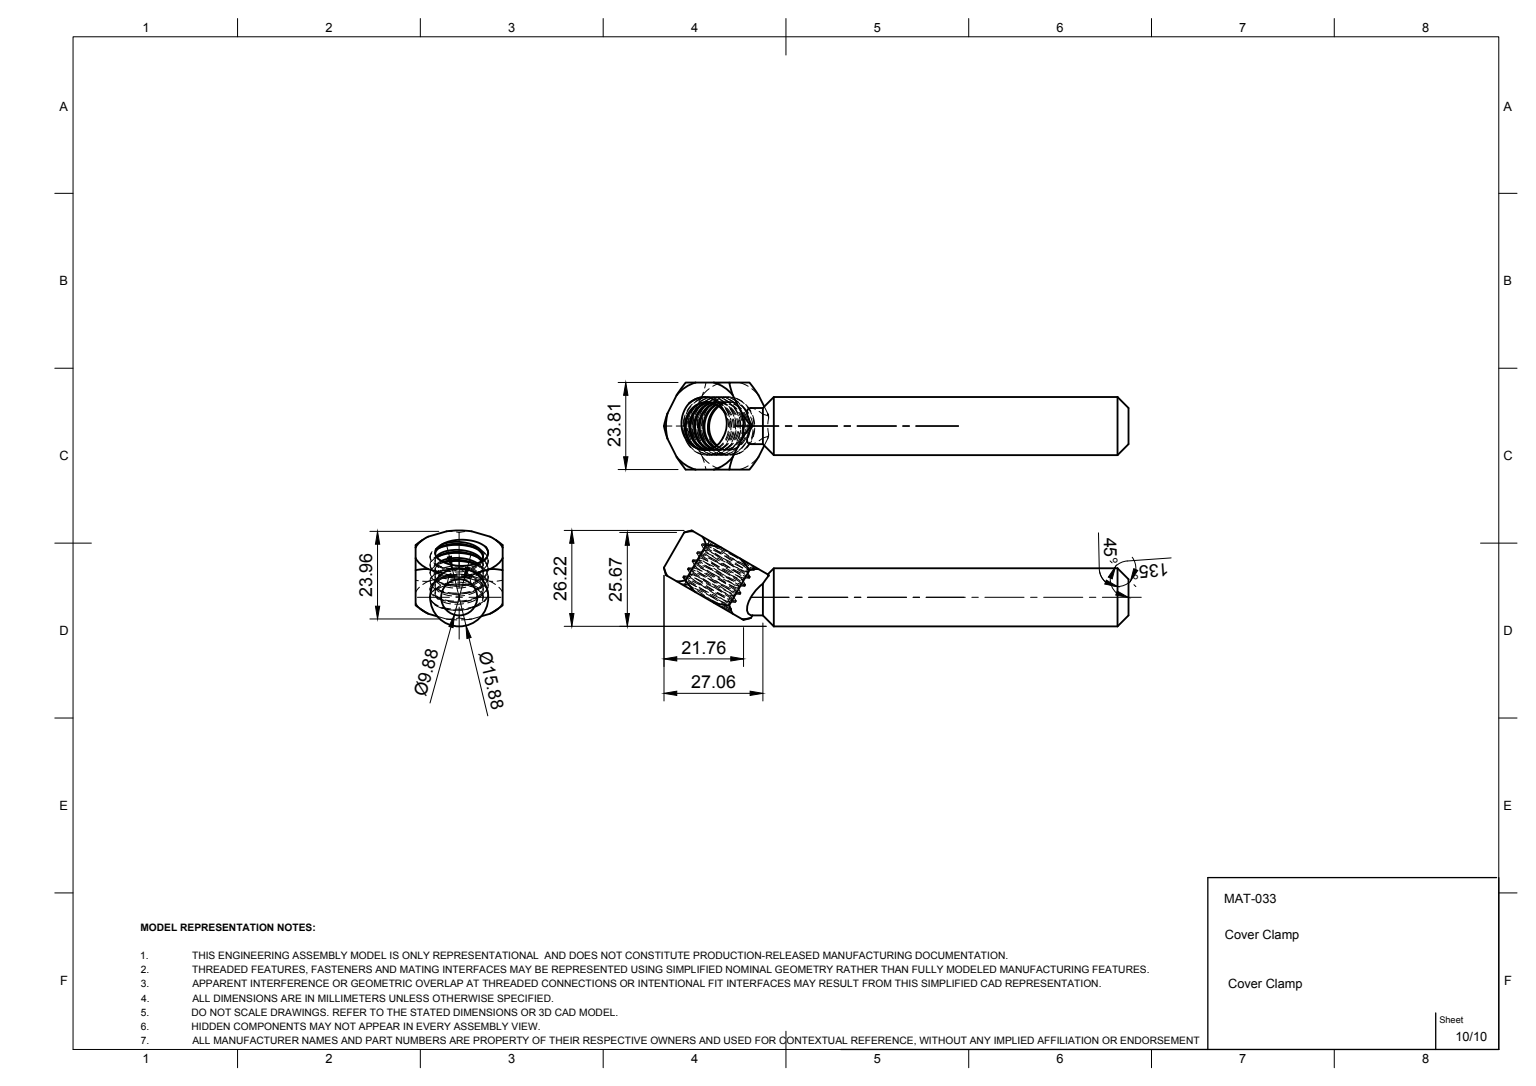
ISO-10303-21;
HEADER;
/* Generated by software containing ST-Developer
 * from STEP Tools, Inc. (www.steptools.com) 
 */

FILE_DESCRIPTION(
/* description */ ('STEP AP214'),
/* implementation_level */ '2;1');

FILE_NAME(
/* name */ 'Cover Clamp.step',
/* time_stamp */ '2026-11-14T07:13:32-08:00',
/* author */ (''),
/* organization */ (''),
/* preprocessor_version */ 'ST-DEVELOPER v20.2',
/* originating_system */ 'Autodesk Translation Framework v15.17.0.0',
/* authorisation */ '');

FILE_SCHEMA (('AUTOMOTIVE_DESIGN { 1 0 10303 214 3 1 1 }'));
ENDSEC;

DATA;
#10=MECHANICAL_DESIGN_GEOMETRIC_PRESENTATION_REPRESENTATION('',(#1323),#32903);
#315=(
BOUNDED_SURFACE()
B_SPLINE_SURFACE(1,2,((#30077,#30078,#30079,#30080,#30081,#30082,#30083,
#30084,#30085,#30086,#30087,#30088,#30089,#30090,#30091,#30092,#30093,#30094,
#30095,#30096,#30097,#30098,#30099,#30100,#30101,#30102,#30103,#30104,#30105,
#30106,#30107,#30108,#30109,#30110,#30111,#30112,#30113,#30114,#30115,#30116,
#30117,#30118,#30119,#30120,#30121,#30122,#30123,#30124,#30125,#30126,#30127,
#30128,#30129,#30130,#30131,#30132,#30133,#30134,#30135,#30136,#30137,#30138,
#30139,#30140,#30141,#30142,#30143,#30144,#30145,#30146,#30147,#30148,#30149,
#30150,#30151,#30152,#30153,#30154,#30155,#30156,#30157,#30158,#30159,#30160,
#30161,#30162,#30163,#30164,#30165,#30166,#30167,#30168,#30169,#30170,#30171,
#30172,#30173,#30174,#30175,#30176,#30177,#30178,#30179,#30180,#30181,#30182,
#30183,#30184,#30185,#30186,#30187,#30188,#30189,#30190,#30191,#30192,#30193,
#30194,#30195,#30196,#30197,#30198,#30199,#30200,#30201,#30202,#30203,#30204,
#30205,#30206,#30207,#30208,#30209,#30210,#30211,#30212,#30213),(#30214,
#30215,#30216,#30217,#30218,#30219,#30220,#30221,#30222,#30223,#30224,#30225,
#30226,#30227,#30228,#30229,#30230,#30231,#30232,#30233,#30234,#30235,#30236,
#30237,#30238,#30239,#30240,#30241,#30242,#30243,#30244,#30245,#30246,#30247,
#30248,#30249,#30250,#30251,#30252,#30253,#30254,#30255,#30256,#30257,#30258,
#30259,#30260,#30261,#30262,#30263,#30264,#30265,#30266,#30267,#30268,#30269,
#30270,#30271,#30272,#30273,#30274,#30275,#30276,#30277,#30278,#30279,#30280,
#30281,#30282,#30283,#30284,#30285,#30286,#30287,#30288,#30289,#30290,#30291,
#30292,#30293,#30294,#30295,#30296,#30297,#30298,#30299,#30300,#30301,#30302,
#30303,#30304,#30305,#30306,#30307,#30308,#30309,#30310,#30311,#30312,#30313,
#30314,#30315,#30316,#30317,#30318,#30319,#30320,#30321,#30322,#30323,#30324,
#30325,#30326,#30327,#30328,#30329,#30330,#30331,#30332,#30333,#30334,#30335,
#30336,#30337,#30338,#30339,#30340,#30341,#30342,#30343,#30344,#30345,#30346,
#30347,#30348,#30349,#30350)),.UNSPECIFIED.,.F.,.F.,.F.)
B_SPLINE_SURFACE_WITH_KNOTS((2,2),(3,2,2,2,2,2,2,2,2,2,2,2,2,2,2,2,2,2,
2,2,2,2,2,2,2,2,2,2,2,2,2,2,2,2,2,2,2,2,2,2,2,2,2,2,2,2,2,2,2,2,2,2,2,2,
2,2,2,2,2,2,2,2,2,2,2,2,2,2,3),(0.,1.),(0.,0.0142857142857143,0.0285714285714286,
0.0428571428571429,0.0571428571428571,0.0714285714285714,0.0857142857142857,
0.1,0.114285714285714,0.128571428571429,0.142857142857143,0.157142857142857,
0.171428571428571,0.185714285714286,0.2,0.214285714285714,0.228571428571429,
0.242857142857143,0.257142857142857,0.271428571428571,0.285714285714286,
0.3,0.314285714285714,0.328571428571429,0.342857142857143,0.357142857142857,
0.371428571428571,0.385714285714286,0.4,0.414285714285714,0.428571428571429,
0.442857142857143,0.457142857142857,0.471428571428571,0.485714285714286,
0.5,0.514285714285714,0.528571428571429,0.542857142857143,0.557142857142857,
0.571428571428571,0.585714285714286,0.6,0.614285714285714,0.628571428571429,
0.642857142857143,0.657142857142857,0.671428571428571,0.685714285714286,
0.7,0.714285714285714,0.728571428571429,0.742857142857143,0.757142857142857,
0.771428571428571,0.785714285714286,0.8,0.814285714285714,0.828571428571429,
0.842857142857143,0.857142857142857,0.871428571428571,0.885714285714286,
0.9,0.914285714285714,0.928571428571429,0.942857142857143,0.957142857142857,
0.961773175750461),.UNSPECIFIED.)
GEOMETRIC_REPRESENTATION_ITEM()
RATIONAL_B_SPLINE_SURFACE(((1.,0.951056516295154,1.,0.951056516295154,1.,
0.951056516295154,1.,0.951056516295154,1.,0.951056516295154,1.,0.951056516295154,
1.,0.951056516295154,1.,0.951056516295154,1.,0.951056516295154,1.,0.951056516295154,
1.,0.951056516295154,1.,0.951056516295154,1.,0.951056516295154,1.,0.951056516295154,
1.,0.951056516295154,1.,0.951056516295154,1.,0.951056516295154,1.,0.951056516295154,
1.,0.951056516295154,1.,0.951056516295154,1.,0.951056516295154,1.,0.951056516295154,
1.,0.951056516295154,1.,0.951056516295154,1.,0.951056516295154,1.,0.951056516295154,
1.,0.951056516295154,1.,0.951056516295154,1.,0.951056516295154,1.,0.951056516295154,
1.,0.951056516295154,1.,0.951056516295154,1.,0.951056516295154,1.,0.951056516295154,
1.,0.951056516295154,1.,0.951056516295154,1.,0.951056516295154,1.,0.951056516295154,
1.,0.951056516295154,1.,0.951056516295154,1.,0.951056516295154,1.,0.951056516295154,
1.,0.951056516295154,1.,0.951056516295154,1.,0.951056516295154,1.,0.951056516295154,
1.,0.951056516295154,1.,0.951056516295154,1.,0.951056516295154,1.,0.951056516295154,
1.,0.951056516295154,1.,0.951056516295154,1.,0.951056516295154,1.,0.951056516295154,
1.,0.951056516295154,1.,0.951056516295154,1.,0.951056516295154,1.,0.951056516295154,
1.,0.951056516295154,1.,0.951056516295154,1.,0.951056516295154,1.,0.951056516295154,
1.,0.951056516295154,1.,0.951056516295154,1.,0.951056516295154,1.,0.951056516295154,
1.,0.951056516295154,1.,0.984136325367634,0.978556192232199),(1.,0.951056516295154,
1.,0.951056516295154,1.,0.951056516295154,1.,0.951056516295154,1.,0.951056516295154,
1.,0.951056516295154,1.,0.951056516295154,1.,0.951056516295154,1.,0.951056516295154,
1.,0.951056516295154,1.,0.951056516295154,1.,0.951056516295154,1.,0.951056516295154,
1.,0.951056516295154,1.,0.951056516295154,1.,0.951056516295154,1.,0.951056516295154,
1.,0.951056516295154,1.,0.951056516295154,1.,0.951056516295154,1.,0.951056516295154,
1.,0.951056516295154,1.,0.951056516295154,1.,0.951056516295154,1.,0.951056516295154,
1.,0.951056516295154,1.,0.951056516295154,1.,0.951056516295154,1.,0.951056516295154,
1.,0.951056516295154,1.,0.951056516295154,1.,0.951056516295154,1.,0.951056516295154,
1.,0.951056516295154,1.,0.951056516295154,1.,0.951056516295154,1.,0.951056516295154,
1.,0.951056516295154,1.,0.951056516295154,1.,0.951056516295154,1.,0.951056516295154,
1.,0.951056516295154,1.,0.951056516295154,1.,0.951056516295154,1.,0.951056516295154,
1.,0.951056516295154,1.,0.951056516295154,1.,0.951056516295154,1.,0.951056516295154,
1.,0.951056516295154,1.,0.951056516295154,1.,0.951056516295154,1.,0.951056516295154,
1.,0.951056516295154,1.,0.951056516295154,1.,0.951056516295154,1.,0.951056516295154,
1.,0.951056516295154,1.,0.951056516295154,1.,0.951056516295154,1.,0.951056516295154,
1.,0.951056516295154,1.,0.951056516295154,1.,0.951056516295154,1.,0.951056516295154,
1.,0.951056516295154,1.,0.951056516295154,1.,0.984136325367634,0.978556192232199)))
REPRESENTATION_ITEM('')
SURFACE()
);
#316=(
BOUNDED_SURFACE()
B_SPLINE_SURFACE(1,2,((#30394,#30395,#30396,#30397,#30398,#30399,#30400,
#30401,#30402,#30403,#30404,#30405,#30406,#30407,#30408,#30409,#30410,#30411,
#30412,#30413,#30414,#30415,#30416,#30417,#30418,#30419,#30420,#30421,#30422,
#30423,#30424,#30425,#30426,#30427,#30428,#30429,#30430,#30431,#30432,#30433,
#30434,#30435,#30436,#30437,#30438,#30439,#30440,#30441,#30442,#30443,#30444,
#30445,#30446,#30447,#30448,#30449,#30450,#30451,#30452,#30453,#30454,#30455,
#30456,#30457,#30458,#30459,#30460,#30461,#30462,#30463,#30464,#30465,#30466,
#30467,#30468,#30469,#30470,#30471,#30472,#30473,#30474,#30475,#30476,#30477,
#30478,#30479,#30480,#30481,#30482,#30483,#30484,#30485,#30486,#30487,#30488,
#30489,#30490,#30491,#30492,#30493,#30494,#30495,#30496,#30497,#30498,#30499,
#30500,#30501,#30502,#30503,#30504,#30505,#30506,#30507,#30508,#30509,#30510,
#30511,#30512,#30513,#30514,#30515,#30516,#30517,#30518,#30519,#30520,#30521,
#30522,#30523,#30524,#30525,#30526,#30527,#30528,#30529,#30530),(#30531,
#30532,#30533,#30534,#30535,#30536,#30537,#30538,#30539,#30540,#30541,#30542,
#30543,#30544,#30545,#30546,#30547,#30548,#30549,#30550,#30551,#30552,#30553,
#30554,#30555,#30556,#30557,#30558,#30559,#30560,#30561,#30562,#30563,#30564,
#30565,#30566,#30567,#30568,#30569,#30570,#30571,#30572,#30573,#30574,#30575,
#30576,#30577,#30578,#30579,#30580,#30581,#30582,#30583,#30584,#30585,#30586,
#30587,#30588,#30589,#30590,#30591,#30592,#30593,#30594,#30595,#30596,#30597,
#30598,#30599,#30600,#30601,#30602,#30603,#30604,#30605,#30606,#30607,#30608,
#30609,#30610,#30611,#30612,#30613,#30614,#30615,#30616,#30617,#30618,#30619,
#30620,#30621,#30622,#30623,#30624,#30625,#30626,#30627,#30628,#30629,#30630,
#30631,#30632,#30633,#30634,#30635,#30636,#30637,#30638,#30639,#30640,#30641,
#30642,#30643,#30644,#30645,#30646,#30647,#30648,#30649,#30650,#30651,#30652,
#30653,#30654,#30655,#30656,#30657,#30658,#30659,#30660,#30661,#30662,#30663,
#30664,#30665,#30666,#30667)),.UNSPECIFIED.,.F.,.F.,.F.)
B_SPLINE_SURFACE_WITH_KNOTS((2,2),(3,2,2,2,2,2,2,2,2,2,2,2,2,2,2,2,2,2,
2,2,2,2,2,2,2,2,2,2,2,2,2,2,2,2,2,2,2,2,2,2,2,2,2,2,2,2,2,2,2,2,2,2,2,2,
2,2,2,2,2,2,2,2,2,2,2,2,2,2,3),(0.,1.),(0.,0.0142857142857143,0.0285714285714286,
0.0428571428571429,0.0571428571428571,0.0714285714285714,0.0857142857142857,
0.1,0.114285714285714,0.128571428571429,0.142857142857143,0.157142857142857,
0.171428571428571,0.185714285714286,0.2,0.214285714285714,0.228571428571429,
0.242857142857143,0.257142857142857,0.271428571428571,0.285714285714286,
0.3,0.314285714285714,0.328571428571429,0.342857142857143,0.357142857142857,
0.371428571428571,0.385714285714286,0.4,0.414285714285714,0.428571428571429,
0.442857142857143,0.457142857142857,0.471428571428571,0.485714285714286,
0.5,0.514285714285714,0.528571428571429,0.542857142857143,0.557142857142857,
0.571428571428571,0.585714285714286,0.6,0.614285714285714,0.628571428571429,
0.642857142857143,0.657142857142857,0.671428571428571,0.685714285714286,
0.7,0.714285714285714,0.728571428571429,0.742857142857143,0.757142857142857,
0.771428571428571,0.785714285714286,0.8,0.814285714285714,0.828571428571429,
0.842857142857143,0.857142857142857,0.871428571428571,0.885714285714286,
0.9,0.914285714285714,0.928571428571429,0.942857142857143,0.957142857142857,
0.961773131622773),.UNSPECIFIED.)
GEOMETRIC_REPRESENTATION_ITEM()
RATIONAL_B_SPLINE_SURFACE(((1.,0.951056516295154,1.,0.951056516295154,1.,
0.951056516295154,1.,0.951056516295154,1.,0.951056516295154,1.,0.951056516295154,
1.,0.951056516295154,1.,0.951056516295154,1.,0.951056516295154,1.,0.951056516295154,
1.,0.951056516295154,1.,0.951056516295154,1.,0.951056516295154,1.,0.951056516295154,
1.,0.951056516295154,1.,0.951056516295154,1.,0.951056516295154,1.,0.951056516295154,
1.,0.951056516295154,1.,0.951056516295154,1.,0.951056516295154,1.,0.951056516295154,
1.,0.951056516295154,1.,0.951056516295154,1.,0.951056516295154,1.,0.951056516295154,
1.,0.951056516295154,1.,0.951056516295154,1.,0.951056516295154,1.,0.951056516295154,
1.,0.951056516295154,1.,0.951056516295154,1.,0.951056516295154,1.,0.951056516295154,
1.,0.951056516295154,1.,0.951056516295154,1.,0.951056516295154,1.,0.951056516295154,
1.,0.951056516295154,1.,0.951056516295154,1.,0.951056516295154,1.,0.951056516295154,
1.,0.951056516295154,1.,0.951056516295154,1.,0.951056516295154,1.,0.951056516295154,
1.,0.951056516295154,1.,0.951056516295154,1.,0.951056516295154,1.,0.951056516295154,
1.,0.951056516295154,1.,0.951056516295154,1.,0.951056516295154,1.,0.951056516295154,
1.,0.951056516295154,1.,0.951056516295154,1.,0.951056516295154,1.,0.951056516295154,
1.,0.951056516295154,1.,0.951056516295154,1.,0.951056516295154,1.,0.951056516295154,
1.,0.951056516295154,1.,0.951056516295154,1.,0.951056516295154,1.,0.951056516295154,
1.,0.951056516295154,1.,0.98413647655103,0.978556298592283),(1.,0.951056516295154,
1.,0.951056516295154,1.,0.951056516295154,1.,0.951056516295154,1.,0.951056516295154,
1.,0.951056516295154,1.,0.951056516295154,1.,0.951056516295154,1.,0.951056516295154,
1.,0.951056516295154,1.,0.951056516295154,1.,0.951056516295154,1.,0.951056516295154,
1.,0.951056516295154,1.,0.951056516295154,1.,0.951056516295154,1.,0.951056516295154,
1.,0.951056516295154,1.,0.951056516295154,1.,0.951056516295154,1.,0.951056516295154,
1.,0.951056516295154,1.,0.951056516295154,1.,0.951056516295154,1.,0.951056516295154,
1.,0.951056516295154,1.,0.951056516295154,1.,0.951056516295154,1.,0.951056516295154,
1.,0.951056516295154,1.,0.951056516295154,1.,0.951056516295154,1.,0.951056516295154,
1.,0.951056516295154,1.,0.951056516295154,1.,0.951056516295154,1.,0.951056516295154,
1.,0.951056516295154,1.,0.951056516295154,1.,0.951056516295154,1.,0.951056516295154,
1.,0.951056516295154,1.,0.951056516295154,1.,0.951056516295154,1.,0.951056516295154,
1.,0.951056516295154,1.,0.951056516295154,1.,0.951056516295154,1.,0.951056516295154,
1.,0.951056516295154,1.,0.951056516295154,1.,0.951056516295154,1.,0.951056516295154,
1.,0.951056516295154,1.,0.951056516295154,1.,0.951056516295154,1.,0.951056516295154,
1.,0.951056516295154,1.,0.951056516295154,1.,0.951056516295154,1.,0.951056516295154,
1.,0.951056516295154,1.,0.951056516295154,1.,0.951056516295154,1.,0.951056516295154,
1.,0.951056516295154,1.,0.951056516295154,1.,0.98413647655103,0.978556298592283)))
REPRESENTATION_ITEM('')
SURFACE()
);
#388=B_SPLINE_CURVE_WITH_KNOTS('',3,(#29368,#29369,#29370,#29371,#29372,
#29373,#29374,#29375),.UNSPECIFIED.,.F.,.F.,(4,2,2,4),(9.99999998608377E-7,
0.266379961876312,0.531813270515335,0.536353198987997),.UNSPECIFIED.);
#389=B_SPLINE_CURVE_WITH_KNOTS('',3,(#29381,#29382,#29383,#29384,#29385,
#29386,#29387,#29388,#29389,#29390,#29391,#29392,#29393,#29394,#29395,#29396,
#29397,#29398,#29399,#29400,#29401,#29402,#29403,#29404,#29405,#29406,#29407,
#29408,#29409,#29410,#29411,#29412,#29413,#29414,#29415,#29416),
 .UNSPECIFIED.,.F.,.F.,(4,2,2,2,2,2,2,2,2,2,2,2,2,2,2,2,2,4),(22.8834714331197,
22.9155217152857,23.2228277353395,23.5358042737047,23.8457116148797,24.1541920344525,
24.4699609353675,24.7777751890622,25.0888369401879,25.401624583911,25.7090811724736,
26.0228085024749,26.332036183219,26.6411952597108,26.9577480048216,27.265398063477,
27.5359657548391,27.8035129251823),.UNSPECIFIED.);
#390=B_SPLINE_CURVE_WITH_KNOTS('',3,(#29418,#29419,#29420,#29421,#29422,
#29423,#29424,#29425,#29426,#29427,#29428,#29429,#29430,#29431,#29432,#29433,
#29434,#29435,#29436,#29437,#29438,#29439,#29440,#29441,#29442,#29443,#29444,
#29445,#29446,#29447,#29448,#29449,#29450,#29451,#29452,#29453),
 .UNSPECIFIED.,.F.,.F.,(4,2,2,2,2,2,2,2,2,2,2,2,2,2,2,2,2,4),(0.536353198987997,
0.844009151960195,1.15538573983787,1.46301980084842,1.7791232671795,2.0878690803984,
2.39732301411271,2.71061683058146,3.01790845407002,3.33114842108659,3.6418042399083,
3.94969512235302,4.26503959484436,4.57319165957025,4.88342264885394,5.19599272714235,
5.50322598252289,5.5439768298363),.UNSPECIFIED.);
#391=B_SPLINE_CURVE_WITH_KNOTS('',3,(#29458,#29459,#29460,#29461,#29462,
#29463,#29464,#29465,#29466,#29467,#29468,#29469,#29470,#29471,#29472,#29473,
#29474,#29475,#29476,#29477,#29478,#29479,#29480,#29481,#29482,#29483,#29484,
#29485,#29486,#29487,#29488,#29489,#29490,#29491,#29492,#29493),
 .UNSPECIFIED.,.F.,.F.,(4,2,2,2,2,2,2,2,2,2,2,2,2,2,2,2,2,4),(17.8745023500825,
17.9426329487553,18.2502173426604,18.5619029033133,18.8737351023357,19.1814304857963,
19.4958276241938,19.8045434042373,20.1142954786953,20.4295794098716,20.7369298255106,
21.0492181265779,21.360004308523,21.6679912272627,21.983034000075,22.2912070574588,
22.601577623486,22.8834714331197),.UNSPECIFIED.);
#392=B_SPLINE_CURVE_WITH_KNOTS('',3,(#29494,#29495,#29496,#29497,#29498,
#29499,#29500,#29501,#29502,#29503,#29504,#29505,#29506,#29507,#29508,#29509,
#29510,#29511,#29512,#29513,#29514,#29515,#29516,#29517,#29518,#29519,#29520,
#29521,#29522,#29523,#29524,#29525,#29526,#29527,#29528,#29529),
 .UNSPECIFIED.,.F.,.F.,(4,2,2,2,2,2,2,2,2,2,2,2,2,2,2,2,2,4),(5.5439768298363,
5.8177146782931,6.12771125014353,6.43605042222614,6.75070419648573,7.05845758227753,
7.36965133741442,7.68157100910749,7.98894019875319,8.30483846765822,8.61425879594142,
8.92321980318127,9.23727438509702,9.54483326301095,9.85713746478567,10.1685030197442,
10.4761899795599,10.5523964499815),.UNSPECIFIED.);
#393=B_SPLINE_CURVE_WITH_KNOTS('',3,(#29534,#29535,#29536,#29537,#29538,
#29539,#29540,#29541,#29542,#29543,#29544,#29545,#29546,#29547,#29548,#29549,
#29550,#29551,#29552,#29553,#29554,#29555,#29556,#29557,#29558,#29559,#29560,
#29561,#29562,#29563,#29564,#29565,#29566,#29567,#29568,#29569),
 .UNSPECIFIED.,.F.,.F.,(4,2,2,2,2,2,2,2,2,2,2,2,2,2,2,2,2,4),(12.8667522473679,
12.9699770959428,13.2778173876454,13.5932720524022,13.9015013605794,14.2087341790668,
14.5215936127585,14.8314800687057,15.1398530720226,15.4555019865385,15.7632628653506,
16.0742081083735,16.3869911773338,16.694362346664,17.0079690989337,17.3171627992321,
17.6262033882063,17.8745023500825),.UNSPECIFIED.);
#394=B_SPLINE_CURVE_WITH_KNOTS('',3,(#29570,#29571,#29572,#29573,#29574,
#29575,#29576,#29577,#29578,#29579,#29580,#29581,#29582,#29583,#29584,#29585,
#29586,#29587,#29588,#29589,#29590,#29591,#29592,#29593,#29594,#29595,#29596,
#29597,#29598,#29599,#29600,#29601,#29602,#29603,#29604,#29605),
 .UNSPECIFIED.,.F.,.F.,(4,2,2,2,2,2,2,2,2,2,2,2,2,2,2,2,2,4),(10.5523964499815,
10.7922801625917,11.1010192151014,11.4105628806873,11.7238453805044,12.0311675378644,
12.344531578361,12.655179957593,12.9631375944165,13.2784727772684,13.5866311789278,
13.8969661452367,14.2099076813701,14.5197896220926,14.8282363019679,15.1439697099529,
15.4517555491791,15.5606140240025),.UNSPECIFIED.);
#395=B_SPLINE_CURVE_WITH_KNOTS('',3,(#29610,#29611,#29612,#29613,#29614,
#29615,#29616,#29617,#29618,#29619,#29620,#29621,#29622,#29623,#29624,#29625,
#29626,#29627,#29628,#29629,#29630,#29631,#29632,#29633,#29634,#29635,#29636,
#29637,#29638,#29639,#29640,#29641,#29642,#29643,#29644,#29645),
 .UNSPECIFIED.,.F.,.F.,(4,2,2,2,2,2,2,2,2,2,2,2,2,2,2,2,2,4),(7.85839646972881,
7.99675908034552,8.30409236965206,8.61967918417833,8.92922883729377,9.23804955367523,
9.55223789637168,9.85983263591087,10.1718920011921,10.4833809125238,10.790993638598,
11.107215596657,11.4160660862887,11.7254216174803,12.0388290447384,12.3461464639337,
12.6592164371347,12.8667522473679),.UNSPECIFIED.);
#396=B_SPLINE_CURVE_WITH_KNOTS('',3,(#29646,#29647,#29648,#29649,#29650,
#29651,#29652,#29653,#29654,#29655,#29656,#29657,#29658,#29659,#29660,#29661,
#29662,#29663,#29664,#29665,#29666,#29667,#29668,#29669,#29670,#29671,#29672,
#29673,#29674,#29675,#29676,#29677,#29678,#29679,#29680,#29681),
 .UNSPECIFIED.,.F.,.F.,(4,2,2,2,2,2,2,2,2,2,2,2,2,2,2,2,2,4),(15.5606140240025,
15.7627825023106,16.0755461176622,16.3829711914898,16.6966631273082,17.005864177191,
17.3149883873622,17.6315052718071,17.9391257290499,18.2508955674803,18.5627214169535,
18.8704807789836,19.1849651185974,19.4937006141905,19.8035378336403,20.118799733417,
20.4261960881153,20.5702181520879),.UNSPECIFIED.);
#397=B_SPLINE_CURVE_WITH_KNOTS('',3,(#29687,#29688,#29689,#29690,#29691,
#29692,#29693,#29694,#29695,#29696,#29697,#29698,#29699,#29700,#29701,#29702,
#29703,#29704),.UNSPECIFIED.,.F.,.F.,(4,2,2,2,2,2,2,2,4),(25.5798166940227,
25.7130762262509,26.0223265959452,26.3315808307711,26.6482322244482,26.9559321724754,
27.2678326511296,27.5344395661045,27.8029491759931),.UNSPECIFIED.);
#398=B_SPLINE_CURVE_WITH_KNOTS('',3,(#29707,#29708,#29709,#29710,#29711,
#29712,#29713,#29714,#29715,#29716,#29717,#29718,#29719,#29720,#29721,#29722,
#29723,#29724,#29725,#29726,#29727,#29728),.UNSPECIFIED.,.F.,.F.,(4,2,2,
2,2,2,2,2,2,2,4),(0.,0.268131059792874,0.538872031707751,0.846503258776113,
1.15851001858798,1.47006242806841,1.77767654293643,2.09396510009836,2.40287638170031,
2.71219706537191,2.85070864589331),.UNSPECIFIED.);
#399=B_SPLINE_CURVE_WITH_KNOTS('',3,(#29749,#29750,#29751,#29752,#29753,
#29754,#29755),.UNSPECIFIED.,.F.,.F.,(4,3,4),(6.13365413464591E-7,0.000387864803977344,
0.000603704646788277),.UNSPECIFIED.);
#400=B_SPLINE_CURVE_WITH_KNOTS('',3,(#29761,#29762,#29763,#29764,#29765,
#29766,#29767),.UNSPECIFIED.,.F.,.F.,(4,3,4),(0.000817437436689343,0.00120468887525266,
0.00142052871806415),.UNSPECIFIED.);
#401=B_SPLINE_CURVE_WITH_KNOTS('',3,(#29772,#29773,#29774,#29775,#29776,
#29777,#29778,#29779,#29780,#29781,#29782,#29783,#29784,#29785,#29786,#29787,
#29788,#29789,#29790,#29791,#29792,#29793,#29794,#29795,#29796,#29797,#29798,
#29799,#29800,#29801,#29802,#29803,#29804,#29805,#29806,#29807),
 .UNSPECIFIED.,.F.,.F.,(4,2,2,2,2,2,2,2,2,2,2,2,2,2,2,2,2,4),(2.85070864589331,
3.02566872683572,3.33300978172351,3.64601116007675,3.95683190204972,4.26465975012339,
4.5801772316469,4.88845455104737,5.19850753800061,5.51124232253364,5.81848197490562,
6.13269024613722,6.44283634473625,6.75107126604603,7.06588097711394,7.37371520837401,
7.68469288372467,7.85839646972881),.UNSPECIFIED.);
#402=B_SPLINE_CURVE_WITH_KNOTS('',3,(#29808,#29809,#29810,#29811,#29812,
#29813,#29814,#29815,#29816,#29817,#29818,#29819,#29820,#29821,#29822,#29823,
#29824,#29825,#29826,#29827,#29828,#29829,#29830,#29831,#29832,#29833,#29834,
#29835,#29836,#29837,#29838,#29839,#29840,#29841,#29842,#29843),
 .UNSPECIFIED.,.F.,.F.,(4,2,2,2,2,2,2,2,2,2,2,2,2,2,2,2,2,4),(20.5702181520879,
20.7385740104812,21.0493617127615,21.3574237984673,21.6725588611289,21.9807610000102,
22.2912213303042,22.6051519312801,22.9125144828566,23.2255847455386,23.5355035868745,
23.8440698995767,24.1599349233628,24.4677886469063,24.7789436195636,25.0917287398098,
25.3992523291087,25.5798166940227),.UNSPECIFIED.);
#403=B_SPLINE_CURVE_WITH_KNOTS('',3,(#29874,#29875,#29876,#29877),
 .UNSPECIFIED.,.F.,.F.,(4,4),(0.0216842181230129,0.0225335408556301),
 .UNSPECIFIED.);
#404=B_SPLINE_CURVE_WITH_KNOTS('',3,(#29915,#29916,#29917,#29918,#29919,
#29920,#29921,#29922,#29923,#29924,#29925,#29926,#29927,#29928,#29929,#29930,
#29931,#29932,#29933,#29934),.UNSPECIFIED.,.F.,.F.,(4,2,2,2,2,2,2,2,2,4),
(-1.25100528979193,-1.12527766599275,-0.967452239770817,-0.849922888806208,
-0.710459887734631,-0.570917050432261,-0.500208813989938,-0.376689447115683,
-0.191154661349975,0.),.UNSPECIFIED.);
#405=B_SPLINE_CURVE_WITH_KNOTS('',3,(#29935,#29936,#29937,#29938,#29939,
#29940,#29941,#29942,#29943,#29944,#29945,#29946,#29947,#29948,#29949,#29950),
 .UNSPECIFIED.,.F.,.F.,(4,2,2,2,2,2,2,4),(-2.40428630272802,-2.08547605103358,
-1.77189968896946,-1.56153084332572,-0.979972531621945,-0.535421503321372,
-0.245999800540891,0.),.UNSPECIFIED.);
#406=B_SPLINE_CURVE_WITH_KNOTS('',3,(#29970,#29971,#29972,#29973,#29974,
#29975,#29976,#29977,#29978,#29979,#29980,#29981,#29982,#29983),
 .UNSPECIFIED.,.F.,.F.,(4,2,2,2,2,2,4),(0.,0.217946805567693,0.483860386593378,
0.854449493561944,1.0785820352923,1.63181551227744,2.25117072670807),
 .UNSPECIFIED.);
#407=B_SPLINE_CURVE_WITH_KNOTS('',3,(#29984,#29985,#29986,#29987,#29988,
#29989,#29990,#29991,#29992,#29993,#29994,#29995,#29996,#29997,#29998,#29999,
#30000,#30001,#30002,#30003),.UNSPECIFIED.,.F.,.F.,(4,2,2,2,2,2,2,2,2,4),
(0.,0.13295682621977,0.26569932246445,0.351005745590642,0.636655227537102,
0.703754608612356,0.957682580022869,1.06961165453364,1.15307337275592,1.38824210628559),
 .UNSPECIFIED.);
#502=(
BOUNDED_CURVE()
B_SPLINE_CURVE(2,(#29145,#29146,#29147,#29148,#29149,#29150,#29151,#29152,
#29153,#29154,#29155,#29156,#29157,#29158,#29159),.UNSPECIFIED.,.F.,.F.)
B_SPLINE_CURVE_WITH_KNOTS((3,2,2,2,2,2,2,3),(0.816943476460579,0.831796994214408,
0.846650511968236,0.861504029722065,0.876357547475894,0.891211065229723,
0.906064582983552,0.916368765855157),.UNSPECIFIED.)
CURVE()
GEOMETRIC_REPRESENTATION_ITEM()
RATIONAL_B_SPLINE_CURVE((1.,0.951056516295154,1.,0.951056516295154,1.,0.951056516295154,
1.,0.951056516295154,1.,0.951056516295154,1.,0.951056516295154,1.,0.966046924720029,
0.979201706654285))
REPRESENTATION_ITEM('')
);
#503=(
BOUNDED_CURVE()
B_SPLINE_CURVE(2,(#29162,#29163,#29164,#29165,#29166,#29167,#29168,#29169,
#29170,#29171,#29172,#29173,#29174,#29175,#29176,#29177,#29178,#29179,#29180,
#29181,#29182),.UNSPECIFIED.,.F.,.F.)
B_SPLINE_CURVE_WITH_KNOTS((3,2,2,2,2,2,2,2,2,2,3),(0.785714285714286,0.8,
0.814285714285714,0.828571428571429,0.842857142857143,0.857142857142857,
0.871428571428571,0.885714285714286,0.9,0.914285714285714,0.917180190333488),
 .UNSPECIFIED.)
CURVE()
GEOMETRIC_REPRESENTATION_ITEM()
RATIONAL_B_SPLINE_CURVE((1.,0.951056516295154,1.,0.951056516295154,1.,0.951056516295154,
1.,0.951056516295154,1.,0.951056516295154,1.,0.951056516295154,1.,0.951056516295154,
1.,0.951056516295154,1.,0.951056516295154,1.,0.99008339811052,0.984185267551257))
REPRESENTATION_ITEM('')
);
#504=(
BOUNDED_CURVE()
B_SPLINE_CURVE(2,(#29187,#29188,#29189,#29190,#29191,#29192,#29193,#29194,
#29195,#29196,#29197,#29198,#29199,#29200,#29201,#29202,#29203,#29204,#29205,
#29206,#29207),.UNSPECIFIED.,.F.,.F.)
B_SPLINE_CURVE_WITH_KNOTS((3,2,2,2,2,2,2,2,2,2,3),(0.66840829892229,0.683261816676119,
0.698115334429948,0.712968852183777,0.727822369937606,0.742675887691435,
0.757529405445263,0.772382923199092,0.787236440952921,0.80208995870675,
0.816943476460579),.UNSPECIFIED.)
CURVE()
GEOMETRIC_REPRESENTATION_ITEM()
RATIONAL_B_SPLINE_CURVE((1.,0.951056516295154,1.,0.951056516295154,1.,0.951056516295154,
1.,0.951056516295154,1.,0.951056516295154,1.,0.951056516295154,1.,0.951056516295154,
1.,0.951056516295154,1.,0.951056516295154,1.,0.951056516295154,1.))
REPRESENTATION_ITEM('')
);
#505=(
BOUNDED_CURVE()
B_SPLINE_CURVE(2,(#29208,#29209,#29210,#29211,#29212,#29213,#29214,#29215,
#29216,#29217,#29218,#29219,#29220,#29221,#29222,#29223,#29224,#29225,#29226,
#29227,#29228),.UNSPECIFIED.,.F.,.F.)
B_SPLINE_CURVE_WITH_KNOTS((3,2,2,2,2,2,2,2,2,2,3),(0.642857142857143,0.657142857142857,
0.671428571428571,0.685714285714286,0.7,0.714285714285714,0.728571428571429,
0.742857142857143,0.757142857142857,0.771428571428571,0.785714285714286),
 .UNSPECIFIED.)
CURVE()
GEOMETRIC_REPRESENTATION_ITEM()
RATIONAL_B_SPLINE_CURVE((1.,0.951056516295154,1.,0.951056516295154,1.,0.951056516295154,
1.,0.951056516295154,1.,0.951056516295154,1.,0.951056516295154,1.,0.951056516295154,
1.,0.951056516295154,1.,0.951056516295154,1.,0.951056516295154,1.))
REPRESENTATION_ITEM('')
);
#506=(
BOUNDED_CURVE()
B_SPLINE_CURVE(2,(#29233,#29234,#29235,#29236,#29237,#29238,#29239,#29240,
#29241,#29242,#29243,#29244,#29245,#29246,#29247,#29248,#29249,#29250,#29251,
#29252,#29253),.UNSPECIFIED.,.F.,.F.)
B_SPLINE_CURVE_WITH_KNOTS((3,2,2,2,2,2,2,2,2,2,3),(0.519873121384002,0.534726639137831,
0.54958015689166,0.564433674645489,0.579287192399317,0.594140710153146,
0.608994227906975,0.623847745660804,0.638701263414633,0.653554781168462,
0.66840829892229),.UNSPECIFIED.)
CURVE()
GEOMETRIC_REPRESENTATION_ITEM()
RATIONAL_B_SPLINE_CURVE((1.,0.951056516295154,1.,0.951056516295154,1.,0.951056516295154,
1.,0.951056516295154,1.,0.951056516295154,1.,0.951056516295154,1.,0.951056516295154,
1.,0.951056516295154,1.,0.951056516295154,1.,0.951056516295154,1.))
REPRESENTATION_ITEM('')
);
#507=(
BOUNDED_CURVE()
B_SPLINE_CURVE(2,(#29254,#29255,#29256,#29257,#29258,#29259,#29260,#29261,
#29262,#29263,#29264,#29265,#29266,#29267,#29268,#29269,#29270,#29271,#29272,
#29273,#29274),.UNSPECIFIED.,.F.,.F.)
B_SPLINE_CURVE_WITH_KNOTS((3,2,2,2,2,2,2,2,2,2,3),(0.5,0.514285714285714,
0.528571428571429,0.542857142857143,0.557142857142857,0.571428571428571,
0.585714285714286,0.6,0.614285714285714,0.628571428571429,0.642857142857143),
 .UNSPECIFIED.)
CURVE()
GEOMETRIC_REPRESENTATION_ITEM()
RATIONAL_B_SPLINE_CURVE((1.,0.951056516295154,1.,0.951056516295154,1.,0.951056516295154,
1.,0.951056516295154,1.,0.951056516295154,1.,0.951056516295154,1.,0.951056516295154,
1.,0.951056516295154,1.,0.951056516295154,1.,0.951056516295154,1.))
REPRESENTATION_ITEM('')
);
#508=(
BOUNDED_CURVE()
B_SPLINE_CURVE(2,(#29279,#29280,#29281,#29282,#29283,#29284,#29285,#29286,
#29287,#29288,#29289,#29290,#29291,#29292,#29293,#29294,#29295,#29296,#29297,
#29298,#29299),.UNSPECIFIED.,.F.,.F.)
B_SPLINE_CURVE_WITH_KNOTS((3,2,2,2,2,2,2,2,2,2,3),(0.371337943845714,0.386191461599543,
0.401044979353371,0.4158984971072,0.430752014861029,0.445605532614858,0.460459050368687,
0.475312568122516,0.490166085876344,0.505019603630173,0.519873121384002),
 .UNSPECIFIED.)
CURVE()
GEOMETRIC_REPRESENTATION_ITEM()
RATIONAL_B_SPLINE_CURVE((1.,0.951056516295154,1.,0.951056516295154,1.,0.951056516295154,
1.,0.951056516295154,1.,0.951056516295154,1.,0.951056516295154,1.,0.951056516295154,
1.,0.951056516295154,1.,0.951056516295154,1.,0.951056516295154,1.))
REPRESENTATION_ITEM('')
);
#509=(
BOUNDED_CURVE()
B_SPLINE_CURVE(2,(#29300,#29301,#29302,#29303,#29304,#29305,#29306,#29307,
#29308,#29309,#29310,#29311,#29312,#29313,#29314,#29315,#29316,#29317,#29318,
#29319,#29320),.UNSPECIFIED.,.F.,.F.)
B_SPLINE_CURVE_WITH_KNOTS((3,2,2,2,2,2,2,2,2,2,3),(0.357142857142857,0.371428571428571,
0.385714285714286,0.4,0.414285714285714,0.428571428571428,0.442857142857143,
0.457142857142857,0.471428571428571,0.485714285714286,0.5),
 .UNSPECIFIED.)
CURVE()
GEOMETRIC_REPRESENTATION_ITEM()
RATIONAL_B_SPLINE_CURVE((1.,0.951056516295154,1.,0.951056516295154,1.,0.951056516295154,
1.,0.951056516295154,1.,0.951056516295154,1.,0.951056516295154,1.,0.951056516295154,
1.,0.951056516295154,1.,0.951056516295154,1.,0.951056516295154,1.))
REPRESENTATION_ITEM('')
);
#510=(
BOUNDED_CURVE()
B_SPLINE_CURVE(2,(#29326,#29327,#29328,#29329,#29330,#29331,#29332,#29333,
#29334,#29335,#29336,#29337,#29338,#29339,#29340),.UNSPECIFIED.,.F.,.F.)
B_SPLINE_CURVE_WITH_KNOTS((3,2,2,2,2,2,2,3),(0.124029642498174,0.128571428571429,
0.142857142857143,0.157142857142857,0.171428571428571,0.185714285714286,
0.2,0.214285714285714),.UNSPECIFIED.)
CURVE()
GEOMETRIC_REPRESENTATION_ITEM()
RATIONAL_B_SPLINE_CURVE((0.978773338025185,0.984439641713294,1.,0.951056516295154,
1.,0.951056516295154,1.,0.951056516295154,1.,0.951056516295154,1.,0.951056516295154,
1.,0.951056516295154,1.))
REPRESENTATION_ITEM('')
);
#511=(
BOUNDED_CURVE()
B_SPLINE_CURVE(2,(#29343,#29344,#29345,#29346,#29347,#29348,#29349,#29350,
#29351,#29352,#29353,#29354,#29355,#29356,#29357,#29358,#29359,#29360,#29361),
 .UNSPECIFIED.,.F.,.F.)
B_SPLINE_CURVE_WITH_KNOTS((3,2,2,2,2,2,2,2,2,3),(0.091954686099144,0.103974624276795,
0.118828142030624,0.133681659784452,0.148535177538281,0.16338869529211,
0.178242213045939,0.193095730799768,0.207949248553597,0.222802766307425),
 .UNSPECIFIED.)
CURVE()
GEOMETRIC_REPRESENTATION_ITEM()
RATIONAL_B_SPLINE_CURVE((0.984888628507613,0.96039337899068,1.,0.951056516295154,
1.,0.951056516295154,1.,0.951056516295154,1.,0.951056516295154,1.,0.951056516295154,
1.,0.951056516295154,1.,0.951056516295154,1.,0.951056516295154,1.))
REPRESENTATION_ITEM('')
);
#512=(
BOUNDED_CURVE()
B_SPLINE_CURVE(2,(#29757,#29758,#29759),.UNSPECIFIED.,.F.,.F.)
B_SPLINE_CURVE_WITH_KNOTS((3,3),(1.62371575593398,2.33717063536819),
 .UNSPECIFIED.)
CURVE()
GEOMETRIC_REPRESENTATION_ITEM()
RATIONAL_B_SPLINE_CURVE((1.32286062935255,1.34451361022803,1.32286062935255))
REPRESENTATION_ITEM('')
);
#513=(
BOUNDED_CURVE()
B_SPLINE_CURVE(2,(#29846,#29847,#29848),.UNSPECIFIED.,.F.,.F.)
B_SPLINE_CURVE_WITH_KNOTS((3,3),(2.20401193750953,2.35502343804526),
 .UNSPECIFIED.)
CURVE()
GEOMETRIC_REPRESENTATION_ITEM()
RATIONAL_B_SPLINE_CURVE((1.61068751795193,1.61882963884505,1.62522061017657))
REPRESENTATION_ITEM('')
);
#514=(
BOUNDED_CURVE()
B_SPLINE_CURVE(2,(#29856,#29857,#29858),.UNSPECIFIED.,.F.,.F.)
B_SPLINE_CURVE_WITH_KNOTS((3,3),(-2.35502343804526,-1.66463996329892),
 .UNSPECIFIED.)
CURVE()
GEOMETRIC_REPRESENTATION_ITEM()
RATIONAL_B_SPLINE_CURVE((1.62522061017657,1.59600282888702,1.53018480461537))
REPRESENTATION_ITEM('')
);
#515=(
BOUNDED_CURVE()
B_SPLINE_CURVE(2,(#29862,#29863,#29864),.UNSPECIFIED.,.F.,.F.)
B_SPLINE_CURVE_WITH_KNOTS((3,3),(-4.14763863034457,-3.45725829975021),
 .UNSPECIFIED.)
CURVE()
GEOMETRIC_REPRESENTATION_ITEM()
RATIONAL_B_SPLINE_CURVE((1.53017908155183,1.59599685965665,1.62521453166841))
REPRESENTATION_ITEM('')
);
#516=(
BOUNDED_CURVE()
B_SPLINE_CURVE(2,(#29868,#29869,#29870),.UNSPECIFIED.,.F.,.F.)
B_SPLINE_CURVE_WITH_KNOTS((3,3),(-2.35500433297853,-1.66462400238418),
 .UNSPECIFIED.)
CURVE()
GEOMETRIC_REPRESENTATION_ITEM()
RATIONAL_B_SPLINE_CURVE((1.62521453166841,1.59599685965665,1.53017908155183))
REPRESENTATION_ITEM('')
);
#517=(
BOUNDED_CURVE()
B_SPLINE_CURVE(2,(#29880,#29881,#29882),.UNSPECIFIED.,.F.,.F.)
B_SPLINE_CURVE_WITH_KNOTS((3,3),(-4.1476561584474,-3.45727380684988),
 .UNSPECIFIED.)
CURVE()
GEOMETRIC_REPRESENTATION_ITEM()
RATIONAL_B_SPLINE_CURVE((1.53018276023192,1.59600069656826,1.62521843882178))
REPRESENTATION_ITEM('')
);
#518=(
BOUNDED_CURVE()
B_SPLINE_CURVE(2,(#29886,#29887,#29888),.UNSPECIFIED.,.F.,.F.)
B_SPLINE_CURVE_WITH_KNOTS((3,3),(-2.35501661336581,-1.66463426176827),
 .UNSPECIFIED.)
CURVE()
GEOMETRIC_REPRESENTATION_ITEM()
RATIONAL_B_SPLINE_CURVE((1.62521843882178,1.59600069656826,1.53018276023192))
REPRESENTATION_ITEM('')
);
#519=(
BOUNDED_CURVE()
B_SPLINE_CURVE(2,(#29892,#29893,#29894),.UNSPECIFIED.,.F.,.F.)
B_SPLINE_CURVE_WITH_KNOTS((3,3),(-4.14763863034456,-3.45725829975022),
 .UNSPECIFIED.)
CURVE()
GEOMETRIC_REPRESENTATION_ITEM()
RATIONAL_B_SPLINE_CURVE((1.53017908155184,1.59599685965666,1.62521453166842))
REPRESENTATION_ITEM('')
);
#520=(
BOUNDED_CURVE()
B_SPLINE_CURVE(2,(#30008,#30009,#30010),.UNSPECIFIED.,.F.,.F.)
B_SPLINE_CURVE_WITH_KNOTS((3,3),(-4.14765638055873,-3.45727400335158),
 .UNSPECIFIED.)
CURVE()
GEOMETRIC_REPRESENTATION_ITEM()
RATIONAL_B_SPLINE_CURVE((1.53018280684717,1.59600074518857,1.62521848833218))
REPRESENTATION_ITEM('')
);
#521=(
BOUNDED_CURVE()
B_SPLINE_CURVE(2,(#30011,#30012,#30013),.UNSPECIFIED.,.F.,.F.)
B_SPLINE_CURVE_WITH_KNOTS((3,3),(-2.35501676897952,-1.66463439177237),
 .UNSPECIFIED.)
CURVE()
GEOMETRIC_REPRESENTATION_ITEM()
RATIONAL_B_SPLINE_CURVE((1.62521848833218,1.59600074518857,1.53018280684717))
REPRESENTATION_ITEM('')
);
#522=(
BOUNDED_CURVE()
B_SPLINE_CURVE(2,(#30014,#30015,#30016),.UNSPECIFIED.,.F.,.F.)
B_SPLINE_CURVE_WITH_KNOTS((3,3),(-4.14763863034456,-3.45725829975021),
 .UNSPECIFIED.)
CURVE()
GEOMETRIC_REPRESENTATION_ITEM()
RATIONAL_B_SPLINE_CURVE((1.53017908155183,1.59599685965666,1.62521453166841))
REPRESENTATION_ITEM('')
);
#523=(
BOUNDED_CURVE()
B_SPLINE_CURVE(2,(#30017,#30018,#30019),.UNSPECIFIED.,.F.,.F.)
B_SPLINE_CURVE_WITH_KNOTS((3,3),(-2.35500433297852,-1.66462400238418),
 .UNSPECIFIED.)
CURVE()
GEOMETRIC_REPRESENTATION_ITEM()
RATIONAL_B_SPLINE_CURVE((1.62521453166841,1.59599685965665,1.53017908155183))
REPRESENTATION_ITEM('')
);
#524=(
BOUNDED_CURVE()
B_SPLINE_CURVE(2,(#30024,#30025,#30026),.UNSPECIFIED.,.F.,.F.)
B_SPLINE_CURVE_WITH_KNOTS((3,3),(-4.1476658994832,-3.45728242473689),
 .UNSPECIFIED.)
CURVE()
GEOMETRIC_REPRESENTATION_ITEM()
RATIONAL_B_SPLINE_CURVE((1.53018480461537,1.59600282888702,1.62522061017657))
REPRESENTATION_ITEM('')
);
#525=(
BOUNDED_CURVE()
B_SPLINE_CURVE(2,(#30027,#30028,#30029),.UNSPECIFIED.,.F.,.F.)
B_SPLINE_CURVE_WITH_KNOTS((3,3),(-2.35502343804527,-1.66463996329893),
 .UNSPECIFIED.)
CURVE()
GEOMETRIC_REPRESENTATION_ITEM()
RATIONAL_B_SPLINE_CURVE((1.62522061017658,1.59600282888702,1.53018480461537))
REPRESENTATION_ITEM('')
);
#526=(
BOUNDED_CURVE()
B_SPLINE_CURVE(2,(#30030,#30031,#30032),.UNSPECIFIED.,.F.,.F.)
B_SPLINE_CURVE_WITH_KNOTS((3,3),(-4.14763863034457,-3.45725829975024),
 .UNSPECIFIED.)
CURVE()
GEOMETRIC_REPRESENTATION_ITEM()
RATIONAL_B_SPLINE_CURVE((1.53017908155183,1.59599685965666,1.62521453166841))
REPRESENTATION_ITEM('')
);
#527=(
BOUNDED_CURVE()
B_SPLINE_CURVE(2,(#30033,#30034,#30035),.UNSPECIFIED.,.F.,.F.)
B_SPLINE_CURVE_WITH_KNOTS((3,3),(-2.35500433297853,-1.66462400238417),
 .UNSPECIFIED.)
CURVE()
GEOMETRIC_REPRESENTATION_ITEM()
RATIONAL_B_SPLINE_CURVE((1.62521453166842,1.59599685965666,1.53017908155183))
REPRESENTATION_ITEM('')
);
#528=(
BOUNDED_CURVE()
B_SPLINE_CURVE(2,(#30040,#30041,#30042),.UNSPECIFIED.,.F.,.F.)
B_SPLINE_CURVE_WITH_KNOTS((3,3),(-4.14766589948319,-3.45728242473685),
 .UNSPECIFIED.)
CURVE()
GEOMETRIC_REPRESENTATION_ITEM()
RATIONAL_B_SPLINE_CURVE((1.53018480461536,1.59600282888702,1.62522061017657))
REPRESENTATION_ITEM('')
);
#529=(
BOUNDED_CURVE()
B_SPLINE_CURVE(2,(#30043,#30044,#30045),.UNSPECIFIED.,.F.,.F.)
B_SPLINE_CURVE_WITH_KNOTS((3,3),(-2.35502343804525,-1.66463996329893),
 .UNSPECIFIED.)
CURVE()
GEOMETRIC_REPRESENTATION_ITEM()
RATIONAL_B_SPLINE_CURVE((1.62522061017657,1.59600282888702,1.53018480461537))
REPRESENTATION_ITEM('')
);
#530=(
BOUNDED_CURVE()
B_SPLINE_CURVE(2,(#30046,#30047,#30048),.UNSPECIFIED.,.F.,.F.)
B_SPLINE_CURVE_WITH_KNOTS((3,3),(-4.14763863034458,-3.45725829975023),
 .UNSPECIFIED.)
CURVE()
GEOMETRIC_REPRESENTATION_ITEM()
RATIONAL_B_SPLINE_CURVE((1.53017908155183,1.59599685965666,1.62521453166842))
REPRESENTATION_ITEM('')
);
#531=(
BOUNDED_CURVE()
B_SPLINE_CURVE(2,(#30049,#30050,#30051),.UNSPECIFIED.,.F.,.F.)
B_SPLINE_CURVE_WITH_KNOTS((3,3),(-2.35500433297852,-1.66462400238417),
 .UNSPECIFIED.)
CURVE()
GEOMETRIC_REPRESENTATION_ITEM()
RATIONAL_B_SPLINE_CURVE((1.62521453166842,1.59599685965666,1.53017908155183))
REPRESENTATION_ITEM('')
);
#532=(
BOUNDED_CURVE()
B_SPLINE_CURVE(2,(#30053,#30054,#30055),.UNSPECIFIED.,.F.,.F.)
B_SPLINE_CURVE_WITH_KNOTS((3,3),(-4.14765638055869,-3.45727400335153),
 .UNSPECIFIED.)
CURVE()
GEOMETRIC_REPRESENTATION_ITEM()
RATIONAL_B_SPLINE_CURVE((1.53018280684716,1.59600074518856,1.62521848833216))
REPRESENTATION_ITEM('')
);
#533=(
BOUNDED_CURVE()
B_SPLINE_CURVE(2,(#30056,#30057,#30058),.UNSPECIFIED.,.F.,.F.)
B_SPLINE_CURVE_WITH_KNOTS((3,3),(-2.35501676897951,-1.66463439177237),
 .UNSPECIFIED.)
CURVE()
GEOMETRIC_REPRESENTATION_ITEM()
RATIONAL_B_SPLINE_CURVE((1.62521848833216,1.59600074518856,1.53018280684716))
REPRESENTATION_ITEM('')
);
#534=(
BOUNDED_CURVE()
B_SPLINE_CURVE(2,(#30059,#30060,#30061),.UNSPECIFIED.,.F.,.F.)
B_SPLINE_CURVE_WITH_KNOTS((3,3),(-4.14763863034457,-3.45725829975022),
 .UNSPECIFIED.)
CURVE()
GEOMETRIC_REPRESENTATION_ITEM()
RATIONAL_B_SPLINE_CURVE((1.53017908155183,1.59599685965666,1.62521453166842))
REPRESENTATION_ITEM('')
);
#535=(
BOUNDED_CURVE()
B_SPLINE_CURVE(2,(#30062,#30063,#30064),.UNSPECIFIED.,.F.,.F.)
B_SPLINE_CURVE_WITH_KNOTS((3,3),(-2.35500433297853,-1.66462400238418),
 .UNSPECIFIED.)
CURVE()
GEOMETRIC_REPRESENTATION_ITEM()
RATIONAL_B_SPLINE_CURVE((1.62521453166842,1.59599685965666,1.53017908155183))
REPRESENTATION_ITEM('')
);
#536=(
BOUNDED_CURVE()
B_SPLINE_CURVE(2,(#30351,#30352,#30353,#30354,#30355,#30356,#30357,#30358,
#30359,#30360,#30361,#30362,#30363,#30364,#30365,#30366,#30367,#30368,#30369,
#30370,#30371),.UNSPECIFIED.,.F.,.F.)
B_SPLINE_CURVE_WITH_KNOTS((3,2,2,2,2,2,2,2,2,2,3),(0.214285714285714,0.228571428571429,
0.242857142857143,0.257142857142857,0.271428571428571,0.285714285714286,
0.3,0.314285714285714,0.328571428571429,0.342857142857143,0.357142857142857),
 .UNSPECIFIED.)
CURVE()
GEOMETRIC_REPRESENTATION_ITEM()
RATIONAL_B_SPLINE_CURVE((1.,0.951056516295154,1.,0.951056516295154,1.,0.951056516295154,
1.,0.951056516295154,1.,0.951056516295154,1.,0.951056516295154,1.,0.951056516295154,
1.,0.951056516295154,1.,0.951056516295154,1.,0.951056516295154,1.))
REPRESENTATION_ITEM('')
);
#537=(
BOUNDED_CURVE()
B_SPLINE_CURVE(2,(#30373,#30374,#30375,#30376,#30377,#30378,#30379,#30380,
#30381,#30382,#30383,#30384,#30385,#30386,#30387,#30388,#30389,#30390,#30391,
#30392,#30393),.UNSPECIFIED.,.F.,.F.)
B_SPLINE_CURVE_WITH_KNOTS((3,2,2,2,2,2,2,2,2,2,3),(0.222802766307425,0.237656284061254,
0.252509801815083,0.267363319568912,0.282216837322741,0.29707035507657,
0.311923872830398,0.326777390584227,0.341630908338056,0.356484426091885,
0.371337943845714),.UNSPECIFIED.)
CURVE()
GEOMETRIC_REPRESENTATION_ITEM()
RATIONAL_B_SPLINE_CURVE((1.,0.951056516295154,1.,0.951056516295154,1.,0.951056516295154,
1.,0.951056516295154,1.,0.951056516295154,1.,0.951056516295154,1.,0.951056516295154,
1.,0.951056516295154,1.,0.951056516295154,1.,0.951056516295154,1.))
REPRESENTATION_ITEM('')
);
#603=CONICAL_SURFACE('',#16468,4.93749999999997,0.785398163397445);
#604=CONICAL_SURFACE('',#16474,7.9375,0.785398163397451);
#605=CONICAL_SURFACE('',#16480,12.246709909405,0.785398163397453);
#606=CONICAL_SURFACE('',#16504,13.746709909405,0.785398163397448);
#607=CONICAL_SURFACE('',#16505,13.746709909405,0.785398163397448);
#608=CONICAL_SURFACE('',#16506,12.246709909405,0.785398163397453);
#609=CONICAL_SURFACE('',#16507,12.246709909405,0.785398163397453);
#610=CONICAL_SURFACE('',#16508,13.746709909405,0.785398163397448);
#611=CONICAL_SURFACE('',#16509,12.246709909405,0.785398163397453);
#612=CONICAL_SURFACE('',#16510,13.746709909405,0.785398163397448);
#613=CONICAL_SURFACE('',#16511,12.246709909405,0.785398163397453);
#614=CONICAL_SURFACE('',#16512,13.746709909405,0.785398163397448);
#615=CONICAL_SURFACE('',#16513,12.246709909405,0.785398163397453);
#616=CONICAL_SURFACE('',#16514,13.746709909405,0.785398163397448);
#617=CONICAL_SURFACE('',#16515,12.246709909405,0.785398163397453);
#668=ELLIPSE('',#16476,29.6250000052051,10.4740191977281);
#669=ELLIPSE('',#16477,29.6250000012,10.4740191966556);
#670=ELLIPSE('',#16483,6.58333333333336,4.93750000000003);
#671=ELLIPSE('',#16485,6.58333333333341,4.93750000000007);
#680=SHAPE_REPRESENTATION_RELATIONSHIP('SRR','None',#33022,#694);
#694=ADVANCED_BREP_SHAPE_REPRESENTATION('',(#1412),#32897);
#941=CIRCLE('',#16453,6.56268467749995);
#942=CIRCLE('',#16458,6.56268467749995);
#943=CIRCLE('',#16460,7.9375);
#944=CIRCLE('',#16462,7.9375);
#945=CIRCLE('',#16467,7.9375);
#946=CIRCLE('',#16469,7.9375);
#947=CIRCLE('',#16470,4.93749999999997);
#948=CIRCLE('',#16472,7.9375);
#949=CIRCLE('',#16473,7.9375);
#950=CIRCLE('',#16475,4.93750000000002);
#951=CIRCLE('',#16478,4.93750000000002);
#952=CIRCLE('',#16481,12.246709909405);
#953=CIRCLE('',#16487,12.246709909405);
#954=CIRCLE('',#16488,12.246709909405);
#955=CIRCLE('',#16489,12.246709909405);
#956=CIRCLE('',#16490,12.246709909405);
#957=CIRCLE('',#16491,12.246709909405);
#958=CIRCLE('',#16492,12.246709909405);
#959=CIRCLE('',#16494,12.246709909405);
#960=CIRCLE('',#16495,12.246709909405);
#961=CIRCLE('',#16496,12.246709909405);
#962=CIRCLE('',#16497,12.246709909405);
#963=CIRCLE('',#16498,12.246709909405);
#964=CIRCLE('',#16499,12.246709909405);
#1233=CYLINDRICAL_SURFACE('',#16452,6.56268467749995);
#1234=CYLINDRICAL_SURFACE('',#16454,6.56268467749995);
#1235=CYLINDRICAL_SURFACE('',#16455,6.56268467749995);
#1236=CYLINDRICAL_SURFACE('',#16456,6.56268467749995);
#1237=CYLINDRICAL_SURFACE('',#16457,6.56268467749995);
#1238=CYLINDRICAL_SURFACE('',#16459,7.9375);
#1239=CYLINDRICAL_SURFACE('',#16461,7.9375);
#1240=CYLINDRICAL_SURFACE('',#16463,7.9375);
#1241=CYLINDRICAL_SURFACE('',#16464,7.9375);
#1242=CYLINDRICAL_SURFACE('',#16465,7.9375);
#1243=CYLINDRICAL_SURFACE('',#16466,7.9375);
#1244=CYLINDRICAL_SURFACE('',#16471,7.9375);
#1245=CYLINDRICAL_SURFACE('',#16479,7.9375);
#1246=CYLINDRICAL_SURFACE('',#16516,6.56268467749995);
#1247=CYLINDRICAL_SURFACE('',#16517,4.93750000000002);
#1323=STYLED_ITEM('',(#33100),#1412);
#1412=MANIFOLD_SOLID_BREP('Body1',#15571);
#1601=FACE_BOUND('',#3131,.T.);
#1602=FACE_BOUND('',#3133,.T.);
#2085=FACE_OUTER_BOUND('',#3112,.T.);
#2086=FACE_OUTER_BOUND('',#3113,.T.);
#2087=FACE_OUTER_BOUND('',#3114,.T.);
#2088=FACE_OUTER_BOUND('',#3115,.T.);
#2089=FACE_OUTER_BOUND('',#3116,.T.);
#2090=FACE_OUTER_BOUND('',#3117,.T.);
#2091=FACE_OUTER_BOUND('',#3118,.T.);
#2092=FACE_OUTER_BOUND('',#3119,.T.);
#2093=FACE_OUTER_BOUND('',#3120,.T.);
#2094=FACE_OUTER_BOUND('',#3121,.T.);
#2095=FACE_OUTER_BOUND('',#3122,.T.);
#2096=FACE_OUTER_BOUND('',#3123,.T.);
#2097=FACE_OUTER_BOUND('',#3124,.T.);
#2098=FACE_OUTER_BOUND('',#3125,.T.);
#2099=FACE_OUTER_BOUND('',#3126,.T.);
#2100=FACE_OUTER_BOUND('',#3127,.T.);
#2101=FACE_OUTER_BOUND('',#3128,.T.);
#2102=FACE_OUTER_BOUND('',#3129,.T.);
#2103=FACE_OUTER_BOUND('',#3130,.T.);
#2104=FACE_OUTER_BOUND('',#3132,.T.);
#2105=FACE_OUTER_BOUND('',#3134,.T.);
#2106=FACE_OUTER_BOUND('',#3135,.T.);
#2107=FACE_OUTER_BOUND('',#3136,.T.);
#2108=FACE_OUTER_BOUND('',#3137,.T.);
#2109=FACE_OUTER_BOUND('',#3138,.T.);
#2110=FACE_OUTER_BOUND('',#3139,.T.);
#2111=FACE_OUTER_BOUND('',#3140,.T.);
#2112=FACE_OUTER_BOUND('',#3141,.T.);
#2113=FACE_OUTER_BOUND('',#3142,.T.);
#2114=FACE_OUTER_BOUND('',#3143,.T.);
#2115=FACE_OUTER_BOUND('',#3144,.T.);
#2116=FACE_OUTER_BOUND('',#3145,.T.);
#2117=FACE_OUTER_BOUND('',#3146,.T.);
#2118=FACE_OUTER_BOUND('',#3147,.T.);
#2119=FACE_OUTER_BOUND('',#3148,.T.);
#2120=FACE_OUTER_BOUND('',#3149,.T.);
#2121=FACE_OUTER_BOUND('',#3150,.T.);
#2122=FACE_OUTER_BOUND('',#3151,.T.);
#2123=FACE_OUTER_BOUND('',#3152,.T.);
#2124=FACE_OUTER_BOUND('',#3153,.T.);
#2125=FACE_OUTER_BOUND('',#3154,.T.);
#3112=EDGE_LOOP('',(#11877,#11878,#11879,#11880));
#3113=EDGE_LOOP('',(#11881,#11882,#11883,#11884));
#3114=EDGE_LOOP('',(#11885,#11886,#11887,#11888));
#3115=EDGE_LOOP('',(#11889,#11890,#11891,#11892));
#3116=EDGE_LOOP('',(#11893,#11894,#11895,#11896));
#3117=EDGE_LOOP('',(#11897,#11898,#11899));
#3118=EDGE_LOOP('',(#11900,#11901,#11902,#11903,#11904));
#3119=EDGE_LOOP('',(#11905,#11906,#11907,#11908));
#3120=EDGE_LOOP('',(#11909,#11910,#11911,#11912));
#3121=EDGE_LOOP('',(#11913,#11914,#11915,#11916));
#3122=EDGE_LOOP('',(#11917,#11918,#11919,#11920));
#3123=EDGE_LOOP('',(#11921,#11922,#11923,#11924));
#3124=EDGE_LOOP('',(#11925,#11926,#11927,#11928,#11929));
#3125=EDGE_LOOP('',(#11930,#11931,#11932,#11933,#11934,#11935,#11936,#11937,
#11938,#11939,#11940));
#3126=EDGE_LOOP('',(#11941,#11942,#11943,#11944));
#3127=EDGE_LOOP('',(#11945,#11946,#11947));
#3128=EDGE_LOOP('',(#11948,#11949,#11950,#11951,#11952,#11953,#11954,#11955,
#11956,#11957));
#3129=EDGE_LOOP('',(#11958,#11959,#11960,#11961,#11962,#11963,#11964,#11965,
#11966,#11967));
#3130=EDGE_LOOP('',(#11968,#11969,#11970,#11971,#11972,#11973,#11974,#11975,
#11976,#11977,#11978,#11979,#11980,#11981));
#3131=EDGE_LOOP('',(#11982,#11983,#11984,#11985));
#3132=EDGE_LOOP('',(#11986,#11987,#11988,#11989,#11990,#11991,#11992,#11993,
#11994,#11995,#11996,#11997));
#3133=EDGE_LOOP('',(#11998,#11999,#12000,#12001,#12002));
#3134=EDGE_LOOP('',(#12003,#12004,#12005,#12006,#12007,#12008,#12009,#12010));
#3135=EDGE_LOOP('',(#12011,#12012,#12013,#12014,#12015,#12016,#12017,#12018));
#3136=EDGE_LOOP('',(#12019,#12020,#12021,#12022,#12023,#12024,#12025,#12026));
#3137=EDGE_LOOP('',(#12027,#12028,#12029,#12030,#12031,#12032,#12033,#12034));
#3138=EDGE_LOOP('',(#12035,#12036,#12037));
#3139=EDGE_LOOP('',(#12038,#12039,#12040));
#3140=EDGE_LOOP('',(#12041,#12042,#12043));
#3141=EDGE_LOOP('',(#12044,#12045,#12046));
#3142=EDGE_LOOP('',(#12047,#12048,#12049));
#3143=EDGE_LOOP('',(#12050,#12051,#12052));
#3144=EDGE_LOOP('',(#12053,#12054,#12055));
#3145=EDGE_LOOP('',(#12056,#12057,#12058));
#3146=EDGE_LOOP('',(#12059,#12060,#12061));
#3147=EDGE_LOOP('',(#12062,#12063,#12064));
#3148=EDGE_LOOP('',(#12065,#12066,#12067));
#3149=EDGE_LOOP('',(#12068,#12069,#12070));
#3150=EDGE_LOOP('',(#12071,#12072,#12073,#12074,#12075,#12076,#12077,#12078,
#12079,#12080,#12081,#12082,#12083,#12084));
#3151=EDGE_LOOP('',(#12085,#12086,#12087,#12088));
#3152=EDGE_LOOP('',(#12089,#12090,#12091,#12092,#12093,#12094,#12095,#12096,
#12097,#12098,#12099,#12100,#12101,#12102,#12103));
#3153=EDGE_LOOP('',(#12104,#12105,#12106,#12107));
#3154=EDGE_LOOP('',(#12108));
#4228=LINE('',#29143,#5632);
#4229=LINE('',#29186,#5633);
#4230=LINE('',#29232,#5634);
#4231=LINE('',#29278,#5635);
#4232=LINE('',#29324,#5636);
#4233=LINE('',#29365,#5637);
#4234=LINE('',#29379,#5638);
#4235=LINE('',#29457,#5639);
#4236=LINE('',#29533,#5640);
#4237=LINE('',#29609,#5641);
#4238=LINE('',#29685,#5642);
#4239=LINE('',#29733,#5643);
#4240=LINE('',#29739,#5644);
#4241=LINE('',#29743,#5645);
#4242=LINE('',#29854,#5646);
#4243=LINE('',#29860,#5647);
#4244=LINE('',#29866,#5648);
#4245=LINE('',#29871,#5649);
#4246=LINE('',#29884,#5650);
#4247=LINE('',#29890,#5651);
#4248=LINE('',#29895,#5652);
#4249=LINE('',#29901,#5653);
#4250=LINE('',#29905,#5654);
#4251=LINE('',#29909,#5655);
#4252=LINE('',#29913,#5656);
#4253=LINE('',#29955,#5657);
#4254=LINE('',#29959,#5658);
#4255=LINE('',#29963,#5659);
#4256=LINE('',#29967,#5660);
#4257=LINE('',#30007,#5661);
#4258=LINE('',#30023,#5662);
#4259=LINE('',#30039,#5663);
#5632=VECTOR('',#19052,6.56268467749995);
#5633=VECTOR('',#19057,6.56268467749995);
#5634=VECTOR('',#19060,6.56268467749995);
#5635=VECTOR('',#19063,6.56268467749995);
#5636=VECTOR('',#19066,6.56268467749995);
#5637=VECTOR('',#19071,7.9375);
#5638=VECTOR('',#19076,7.9375);
#5639=VECTOR('',#19081,7.9375);
#5640=VECTOR('',#19084,7.9375);
#5641=VECTOR('',#19087,7.9375);
#5642=VECTOR('',#19090,7.9375);
#5643=VECTOR('',#19097,4.93749999999997);
#5644=VECTOR('',#19104,7.9375);
#5645=VECTOR('',#19109,7.9375);
#5646=VECTOR('',#19128,1000.);
#5647=VECTOR('',#19129,1000.);
#5648=VECTOR('',#19130,1000.);
#5649=VECTOR('',#19131,1000.);
#5650=VECTOR('',#19136,1000.);
#5651=VECTOR('',#19137,1000.);
#5652=VECTOR('',#19138,1000.);
#5653=VECTOR('',#19145,1000.);
#5654=VECTOR('',#19148,1000.);
#5655=VECTOR('',#19151,1000.);
#5656=VECTOR('',#19154,1000.);
#5657=VECTOR('',#19161,1000.);
#5658=VECTOR('',#19164,1000.);
#5659=VECTOR('',#19167,1000.);
#5660=VECTOR('',#19170,1000.);
#5661=VECTOR('',#19177,1000.);
#5662=VECTOR('',#19180,1000.);
#5663=VECTOR('',#19183,1000.);
#7123=VERTEX_POINT('',#29141);
#7124=VERTEX_POINT('',#29142);
#7125=VERTEX_POINT('',#29144);
#7126=VERTEX_POINT('',#29160);
#7127=VERTEX_POINT('',#29184);
#7128=VERTEX_POINT('',#29185);
#7129=VERTEX_POINT('',#29230);
#7130=VERTEX_POINT('',#29231);
#7131=VERTEX_POINT('',#29276);
#7132=VERTEX_POINT('',#29277);
#7133=VERTEX_POINT('',#29322);
#7134=VERTEX_POINT('',#29323);
#7135=VERTEX_POINT('',#29325);
#7136=VERTEX_POINT('',#29341);
#7137=VERTEX_POINT('',#29363);
#7138=VERTEX_POINT('',#29364);
#7139=VERTEX_POINT('',#29366);
#7140=VERTEX_POINT('',#29377);
#7141=VERTEX_POINT('',#29378);
#7142=VERTEX_POINT('',#29380);
#7143=VERTEX_POINT('',#29455);
#7144=VERTEX_POINT('',#29456);
#7145=VERTEX_POINT('',#29531);
#7146=VERTEX_POINT('',#29532);
#7147=VERTEX_POINT('',#29607);
#7148=VERTEX_POINT('',#29608);
#7149=VERTEX_POINT('',#29683);
#7150=VERTEX_POINT('',#29684);
#7151=VERTEX_POINT('',#29686);
#7152=VERTEX_POINT('',#29705);
#7153=VERTEX_POINT('',#29730);
#7154=VERTEX_POINT('',#29732);
#7155=VERTEX_POINT('',#29736);
#7156=VERTEX_POINT('',#29737);
#7157=VERTEX_POINT('',#29742);
#7158=VERTEX_POINT('',#29744);
#7159=VERTEX_POINT('',#29746);
#7160=VERTEX_POINT('',#29748);
#7161=VERTEX_POINT('',#29756);
#7162=VERTEX_POINT('',#29760);
#7163=VERTEX_POINT('',#29768);
#7164=VERTEX_POINT('',#29845);
#7165=VERTEX_POINT('',#29851);
#7166=VERTEX_POINT('',#29853);
#7167=VERTEX_POINT('',#29855);
#7168=VERTEX_POINT('',#29859);
#7169=VERTEX_POINT('',#29861);
#7170=VERTEX_POINT('',#29865);
#7171=VERTEX_POINT('',#29867);
#7172=VERTEX_POINT('',#29873);
#7173=VERTEX_POINT('',#29879);
#7174=VERTEX_POINT('',#29883);
#7175=VERTEX_POINT('',#29885);
#7176=VERTEX_POINT('',#29889);
#7177=VERTEX_POINT('',#29891);
#7178=VERTEX_POINT('',#29898);
#7179=VERTEX_POINT('',#29900);
#7180=VERTEX_POINT('',#29902);
#7181=VERTEX_POINT('',#29904);
#7182=VERTEX_POINT('',#29906);
#7183=VERTEX_POINT('',#29908);
#7184=VERTEX_POINT('',#29910);
#7185=VERTEX_POINT('',#29912);
#7186=VERTEX_POINT('',#29952);
#7187=VERTEX_POINT('',#29954);
#7188=VERTEX_POINT('',#29956);
#7189=VERTEX_POINT('',#29958);
#7190=VERTEX_POINT('',#29960);
#7191=VERTEX_POINT('',#29962);
#7192=VERTEX_POINT('',#29964);
#7193=VERTEX_POINT('',#29966);
#7194=VERTEX_POINT('',#30005);
#7195=VERTEX_POINT('',#30006);
#7196=VERTEX_POINT('',#30021);
#7197=VERTEX_POINT('',#30022);
#7198=VERTEX_POINT('',#30037);
#7199=VERTEX_POINT('',#30038);
#8822=EDGE_CURVE('',#7123,#7124,#4228,.T.);
#8823=EDGE_CURVE('',#7124,#7125,#502,.T.);
#8824=EDGE_CURVE('',#7125,#7126,#941,.T.);
#8825=EDGE_CURVE('',#7123,#7126,#503,.T.);
#8826=EDGE_CURVE('',#7127,#7128,#4229,.T.);
#8827=EDGE_CURVE('',#7128,#7124,#504,.T.);
#8828=EDGE_CURVE('',#7127,#7123,#505,.T.);
#8829=EDGE_CURVE('',#7129,#7130,#4230,.T.);
#8830=EDGE_CURVE('',#7130,#7128,#506,.T.);
#8831=EDGE_CURVE('',#7129,#7127,#507,.T.);
#8832=EDGE_CURVE('',#7131,#7132,#4231,.T.);
#8833=EDGE_CURVE('',#7132,#7130,#508,.T.);
#8834=EDGE_CURVE('',#7131,#7129,#509,.T.);
#8835=EDGE_CURVE('',#7133,#7134,#4232,.T.);
#8836=EDGE_CURVE('',#7135,#7133,#510,.T.);
#8837=EDGE_CURVE('',#7135,#7136,#942,.T.);
#8838=EDGE_CURVE('',#7136,#7134,#511,.T.);
#8839=EDGE_CURVE('',#7137,#7138,#4233,.T.);
#8840=EDGE_CURVE('',#7139,#7138,#943,.T.);
#8841=EDGE_CURVE('',#7137,#7139,#388,.F.);
#8842=EDGE_CURVE('',#7140,#7141,#4234,.T.);
#8843=EDGE_CURVE('',#7141,#7142,#389,.T.);
#8844=EDGE_CURVE('',#7138,#7142,#944,.T.);
#8845=EDGE_CURVE('',#7140,#7137,#390,.F.);
#8846=EDGE_CURVE('',#7143,#7144,#4235,.T.);
#8847=EDGE_CURVE('',#7144,#7141,#391,.T.);
#8848=EDGE_CURVE('',#7143,#7140,#392,.F.);
#8849=EDGE_CURVE('',#7145,#7146,#4236,.T.);
#8850=EDGE_CURVE('',#7146,#7144,#393,.T.);
#8851=EDGE_CURVE('',#7145,#7143,#394,.F.);
#8852=EDGE_CURVE('',#7147,#7148,#4237,.T.);
#8853=EDGE_CURVE('',#7148,#7146,#395,.T.);
#8854=EDGE_CURVE('',#7147,#7145,#396,.F.);
#8855=EDGE_CURVE('',#7149,#7150,#4238,.T.);
#8856=EDGE_CURVE('',#7151,#7149,#397,.F.);
#8857=EDGE_CURVE('',#7151,#7152,#945,.T.);
#8858=EDGE_CURVE('',#7152,#7150,#398,.T.);
#8859=EDGE_CURVE('',#7153,#7153,#946,.T.);
#8860=EDGE_CURVE('',#7153,#7154,#4239,.T.);
#8861=EDGE_CURVE('',#7154,#7154,#947,.T.);
#8862=EDGE_CURVE('',#7155,#7156,#948,.T.);
#8863=EDGE_CURVE('',#7156,#7153,#4240,.T.);
#8864=EDGE_CURVE('',#7156,#7155,#949,.T.);
#8865=EDGE_CURVE('',#7155,#7157,#4241,.T.);
#8866=EDGE_CURVE('',#7158,#7157,#950,.T.);
#8867=EDGE_CURVE('',#7159,#7158,#668,.T.);
#8868=EDGE_CURVE('',#7160,#7159,#399,.T.);
#8869=EDGE_CURVE('',#7160,#7161,#512,.F.);
#8870=EDGE_CURVE('',#7162,#7161,#400,.T.);
#8871=EDGE_CURVE('',#7163,#7162,#669,.T.);
#8872=EDGE_CURVE('',#7157,#7163,#951,.T.);
#8873=EDGE_CURVE('',#7150,#7148,#401,.T.);
#8874=EDGE_CURVE('',#7149,#7147,#402,.F.);
#8875=EDGE_CURVE('',#7162,#7164,#513,.T.);
#8876=EDGE_CURVE('',#7161,#7164,#952,.T.);
#8877=EDGE_CURVE('',#7165,#7163,#670,.T.);
#8878=EDGE_CURVE('',#7166,#7164,#4242,.T.);
#8879=EDGE_CURVE('',#7166,#7167,#514,.T.);
#8880=EDGE_CURVE('',#7167,#7168,#4243,.T.);
#8881=EDGE_CURVE('',#7168,#7169,#515,.T.);
#8882=EDGE_CURVE('',#7169,#7170,#4244,.T.);
#8883=EDGE_CURVE('',#7170,#7171,#516,.T.);
#8884=EDGE_CURVE('',#7165,#7171,#4245,.T.);
#8885=EDGE_CURVE('',#7172,#7159,#403,.T.);
#8886=EDGE_CURVE('',#7158,#7165,#671,.T.);
#8887=EDGE_CURVE('',#7171,#7173,#517,.T.);
#8888=EDGE_CURVE('',#7173,#7174,#4246,.T.);
#8889=EDGE_CURVE('',#7174,#7175,#518,.T.);
#8890=EDGE_CURVE('',#7176,#7175,#4247,.T.);
#8891=EDGE_CURVE('',#7176,#7177,#519,.T.);
#8892=EDGE_CURVE('',#7172,#7177,#4248,.T.);
#8893=EDGE_CURVE('',#7172,#7160,#953,.T.);
#8894=EDGE_CURVE('',#7178,#7177,#954,.T.);
#8895=EDGE_CURVE('',#7178,#7179,#4249,.T.);
#8896=EDGE_CURVE('',#7180,#7179,#955,.T.);
#8897=EDGE_CURVE('',#7180,#7181,#4250,.T.);
#8898=EDGE_CURVE('',#7182,#7181,#956,.T.);
#8899=EDGE_CURVE('',#7182,#7183,#4251,.T.);
#8900=EDGE_CURVE('',#7184,#7183,#957,.T.);
#8901=EDGE_CURVE('',#7184,#7185,#4252,.T.);
#8902=EDGE_CURVE('',#7166,#7185,#958,.T.);
#8903=EDGE_CURVE('',#7136,#7151,#404,.T.);
#8904=EDGE_CURVE('',#7152,#7135,#405,.T.);
#8905=EDGE_CURVE('',#7169,#7186,#959,.T.);
#8906=EDGE_CURVE('',#7187,#7186,#4253,.T.);
#8907=EDGE_CURVE('',#7187,#7188,#960,.T.);
#8908=EDGE_CURVE('',#7189,#7188,#4254,.T.);
#8909=EDGE_CURVE('',#7189,#7190,#961,.T.);
#8910=EDGE_CURVE('',#7191,#7190,#4255,.T.);
#8911=EDGE_CURVE('',#7191,#7192,#962,.T.);
#8912=EDGE_CURVE('',#7193,#7192,#4256,.T.);
#8913=EDGE_CURVE('',#7193,#7174,#963,.T.);
#8914=EDGE_CURVE('',#7173,#7170,#964,.T.);
#8915=EDGE_CURVE('',#7126,#7142,#406,.T.);
#8916=EDGE_CURVE('',#7139,#7125,#407,.T.);
#8917=EDGE_CURVE('',#7194,#7195,#4257,.T.);
#8918=EDGE_CURVE('',#7194,#7179,#520,.T.);
#8919=EDGE_CURVE('',#7178,#7176,#521,.T.);
#8920=EDGE_CURVE('',#7175,#7193,#522,.T.);
#8921=EDGE_CURVE('',#7192,#7195,#523,.T.);
#8922=EDGE_CURVE('',#7196,#7197,#4258,.T.);
#8923=EDGE_CURVE('',#7196,#7181,#524,.T.);
#8924=EDGE_CURVE('',#7180,#7194,#525,.T.);
#8925=EDGE_CURVE('',#7195,#7191,#526,.T.);
#8926=EDGE_CURVE('',#7190,#7197,#527,.T.);
#8927=EDGE_CURVE('',#7198,#7199,#4259,.T.);
#8928=EDGE_CURVE('',#7198,#7183,#528,.T.);
#8929=EDGE_CURVE('',#7182,#7196,#529,.T.);
#8930=EDGE_CURVE('',#7197,#7189,#530,.T.);
#8931=EDGE_CURVE('',#7188,#7199,#531,.T.);
#8932=EDGE_CURVE('',#7167,#7185,#532,.T.);
#8933=EDGE_CURVE('',#7184,#7198,#533,.T.);
#8934=EDGE_CURVE('',#7199,#7187,#534,.T.);
#8935=EDGE_CURVE('',#7186,#7168,#535,.T.);
#8936=EDGE_CURVE('',#7133,#7131,#536,.T.);
#8937=EDGE_CURVE('',#7134,#7132,#537,.T.);
#11877=ORIENTED_EDGE('',*,*,#8822,.T.);
#11878=ORIENTED_EDGE('',*,*,#8823,.T.);
#11879=ORIENTED_EDGE('',*,*,#8824,.T.);
#11880=ORIENTED_EDGE('',*,*,#8825,.F.);
#11881=ORIENTED_EDGE('',*,*,#8826,.T.);
#11882=ORIENTED_EDGE('',*,*,#8827,.T.);
#11883=ORIENTED_EDGE('',*,*,#8822,.F.);
#11884=ORIENTED_EDGE('',*,*,#8828,.F.);
#11885=ORIENTED_EDGE('',*,*,#8829,.T.);
#11886=ORIENTED_EDGE('',*,*,#8830,.T.);
#11887=ORIENTED_EDGE('',*,*,#8826,.F.);
#11888=ORIENTED_EDGE('',*,*,#8831,.F.);
#11889=ORIENTED_EDGE('',*,*,#8832,.T.);
#11890=ORIENTED_EDGE('',*,*,#8833,.T.);
#11891=ORIENTED_EDGE('',*,*,#8829,.F.);
#11892=ORIENTED_EDGE('',*,*,#8834,.F.);
#11893=ORIENTED_EDGE('',*,*,#8835,.F.);
#11894=ORIENTED_EDGE('',*,*,#8836,.F.);
#11895=ORIENTED_EDGE('',*,*,#8837,.T.);
#11896=ORIENTED_EDGE('',*,*,#8838,.T.);
#11897=ORIENTED_EDGE('',*,*,#8839,.T.);
#11898=ORIENTED_EDGE('',*,*,#8840,.F.);
#11899=ORIENTED_EDGE('',*,*,#8841,.F.);
#11900=ORIENTED_EDGE('',*,*,#8842,.T.);
#11901=ORIENTED_EDGE('',*,*,#8843,.T.);
#11902=ORIENTED_EDGE('',*,*,#8844,.F.);
#11903=ORIENTED_EDGE('',*,*,#8839,.F.);
#11904=ORIENTED_EDGE('',*,*,#8845,.F.);
#11905=ORIENTED_EDGE('',*,*,#8846,.T.);
#11906=ORIENTED_EDGE('',*,*,#8847,.T.);
#11907=ORIENTED_EDGE('',*,*,#8842,.F.);
#11908=ORIENTED_EDGE('',*,*,#8848,.F.);
#11909=ORIENTED_EDGE('',*,*,#8849,.T.);
#11910=ORIENTED_EDGE('',*,*,#8850,.T.);
#11911=ORIENTED_EDGE('',*,*,#8846,.F.);
#11912=ORIENTED_EDGE('',*,*,#8851,.F.);
#11913=ORIENTED_EDGE('',*,*,#8852,.T.);
#11914=ORIENTED_EDGE('',*,*,#8853,.T.);
#11915=ORIENTED_EDGE('',*,*,#8849,.F.);
#11916=ORIENTED_EDGE('',*,*,#8854,.F.);
#11917=ORIENTED_EDGE('',*,*,#8855,.F.);
#11918=ORIENTED_EDGE('',*,*,#8856,.F.);
#11919=ORIENTED_EDGE('',*,*,#8857,.T.);
#11920=ORIENTED_EDGE('',*,*,#8858,.T.);
#11921=ORIENTED_EDGE('',*,*,#8859,.F.);
#11922=ORIENTED_EDGE('',*,*,#8860,.T.);
#11923=ORIENTED_EDGE('',*,*,#8861,.F.);
#11924=ORIENTED_EDGE('',*,*,#8860,.F.);
#11925=ORIENTED_EDGE('',*,*,#8862,.T.);
#11926=ORIENTED_EDGE('',*,*,#8863,.T.);
#11927=ORIENTED_EDGE('',*,*,#8859,.T.);
#11928=ORIENTED_EDGE('',*,*,#8863,.F.);
#11929=ORIENTED_EDGE('',*,*,#8864,.T.);
#11930=ORIENTED_EDGE('',*,*,#8862,.F.);
#11931=ORIENTED_EDGE('',*,*,#8865,.T.);
#11932=ORIENTED_EDGE('',*,*,#8866,.F.);
#11933=ORIENTED_EDGE('',*,*,#8867,.F.);
#11934=ORIENTED_EDGE('',*,*,#8868,.F.);
#11935=ORIENTED_EDGE('',*,*,#8869,.T.);
#11936=ORIENTED_EDGE('',*,*,#8870,.F.);
#11937=ORIENTED_EDGE('',*,*,#8871,.F.);
#11938=ORIENTED_EDGE('',*,*,#8872,.F.);
#11939=ORIENTED_EDGE('',*,*,#8865,.F.);
#11940=ORIENTED_EDGE('',*,*,#8864,.F.);
#11941=ORIENTED_EDGE('',*,*,#8855,.T.);
#11942=ORIENTED_EDGE('',*,*,#8873,.T.);
#11943=ORIENTED_EDGE('',*,*,#8852,.F.);
#11944=ORIENTED_EDGE('',*,*,#8874,.F.);
#11945=ORIENTED_EDGE('',*,*,#8875,.F.);
#11946=ORIENTED_EDGE('',*,*,#8870,.T.);
#11947=ORIENTED_EDGE('',*,*,#8876,.T.);
#11948=ORIENTED_EDGE('',*,*,#8877,.T.);
#11949=ORIENTED_EDGE('',*,*,#8871,.T.);
#11950=ORIENTED_EDGE('',*,*,#8875,.T.);
#11951=ORIENTED_EDGE('',*,*,#8878,.F.);
#11952=ORIENTED_EDGE('',*,*,#8879,.T.);
#11953=ORIENTED_EDGE('',*,*,#8880,.T.);
#11954=ORIENTED_EDGE('',*,*,#8881,.T.);
#11955=ORIENTED_EDGE('',*,*,#8882,.T.);
#11956=ORIENTED_EDGE('',*,*,#8883,.T.);
#11957=ORIENTED_EDGE('',*,*,#8884,.F.);
#11958=ORIENTED_EDGE('',*,*,#8885,.T.);
#11959=ORIENTED_EDGE('',*,*,#8867,.T.);
#11960=ORIENTED_EDGE('',*,*,#8886,.T.);
#11961=ORIENTED_EDGE('',*,*,#8884,.T.);
#11962=ORIENTED_EDGE('',*,*,#8887,.T.);
#11963=ORIENTED_EDGE('',*,*,#8888,.T.);
#11964=ORIENTED_EDGE('',*,*,#8889,.T.);
#11965=ORIENTED_EDGE('',*,*,#8890,.F.);
#11966=ORIENTED_EDGE('',*,*,#8891,.T.);
#11967=ORIENTED_EDGE('',*,*,#8892,.F.);
#11968=ORIENTED_EDGE('',*,*,#8869,.F.);
#11969=ORIENTED_EDGE('',*,*,#8893,.F.);
#11970=ORIENTED_EDGE('',*,*,#8892,.T.);
#11971=ORIENTED_EDGE('',*,*,#8894,.F.);
#11972=ORIENTED_EDGE('',*,*,#8895,.T.);
#11973=ORIENTED_EDGE('',*,*,#8896,.F.);
#11974=ORIENTED_EDGE('',*,*,#8897,.T.);
#11975=ORIENTED_EDGE('',*,*,#8898,.F.);
#11976=ORIENTED_EDGE('',*,*,#8899,.T.);
#11977=ORIENTED_EDGE('',*,*,#8900,.F.);
#11978=ORIENTED_EDGE('',*,*,#8901,.T.);
#11979=ORIENTED_EDGE('',*,*,#8902,.F.);
#11980=ORIENTED_EDGE('',*,*,#8878,.T.);
#11981=ORIENTED_EDGE('',*,*,#8876,.F.);
#11982=ORIENTED_EDGE('',*,*,#8857,.F.);
#11983=ORIENTED_EDGE('',*,*,#8903,.F.);
#11984=ORIENTED_EDGE('',*,*,#8837,.F.);
#11985=ORIENTED_EDGE('',*,*,#8904,.F.);
#11986=ORIENTED_EDGE('',*,*,#8905,.T.);
#11987=ORIENTED_EDGE('',*,*,#8906,.F.);
#11988=ORIENTED_EDGE('',*,*,#8907,.T.);
#11989=ORIENTED_EDGE('',*,*,#8908,.F.);
#11990=ORIENTED_EDGE('',*,*,#8909,.T.);
#11991=ORIENTED_EDGE('',*,*,#8910,.F.);
#11992=ORIENTED_EDGE('',*,*,#8911,.T.);
#11993=ORIENTED_EDGE('',*,*,#8912,.F.);
#11994=ORIENTED_EDGE('',*,*,#8913,.T.);
#11995=ORIENTED_EDGE('',*,*,#8888,.F.);
#11996=ORIENTED_EDGE('',*,*,#8914,.T.);
#11997=ORIENTED_EDGE('',*,*,#8882,.F.);
#11998=ORIENTED_EDGE('',*,*,#8840,.T.);
#11999=ORIENTED_EDGE('',*,*,#8844,.T.);
#12000=ORIENTED_EDGE('',*,*,#8915,.F.);
#12001=ORIENTED_EDGE('',*,*,#8824,.F.);
#12002=ORIENTED_EDGE('',*,*,#8916,.F.);
#12003=ORIENTED_EDGE('',*,*,#8917,.F.);
#12004=ORIENTED_EDGE('',*,*,#8918,.T.);
#12005=ORIENTED_EDGE('',*,*,#8895,.F.);
#12006=ORIENTED_EDGE('',*,*,#8919,.T.);
#12007=ORIENTED_EDGE('',*,*,#8890,.T.);
#12008=ORIENTED_EDGE('',*,*,#8920,.T.);
#12009=ORIENTED_EDGE('',*,*,#8912,.T.);
#12010=ORIENTED_EDGE('',*,*,#8921,.T.);
#12011=ORIENTED_EDGE('',*,*,#8922,.F.);
#12012=ORIENTED_EDGE('',*,*,#8923,.T.);
#12013=ORIENTED_EDGE('',*,*,#8897,.F.);
#12014=ORIENTED_EDGE('',*,*,#8924,.T.);
#12015=ORIENTED_EDGE('',*,*,#8917,.T.);
#12016=ORIENTED_EDGE('',*,*,#8925,.T.);
#12017=ORIENTED_EDGE('',*,*,#8910,.T.);
#12018=ORIENTED_EDGE('',*,*,#8926,.T.);
#12019=ORIENTED_EDGE('',*,*,#8927,.F.);
#12020=ORIENTED_EDGE('',*,*,#8928,.T.);
#12021=ORIENTED_EDGE('',*,*,#8899,.F.);
#12022=ORIENTED_EDGE('',*,*,#8929,.T.);
#12023=ORIENTED_EDGE('',*,*,#8922,.T.);
#12024=ORIENTED_EDGE('',*,*,#8930,.T.);
#12025=ORIENTED_EDGE('',*,*,#8908,.T.);
#12026=ORIENTED_EDGE('',*,*,#8931,.T.);
#12027=ORIENTED_EDGE('',*,*,#8880,.F.);
#12028=ORIENTED_EDGE('',*,*,#8932,.T.);
#12029=ORIENTED_EDGE('',*,*,#8901,.F.);
#12030=ORIENTED_EDGE('',*,*,#8933,.T.);
#12031=ORIENTED_EDGE('',*,*,#8927,.T.);
#12032=ORIENTED_EDGE('',*,*,#8934,.T.);
#12033=ORIENTED_EDGE('',*,*,#8906,.T.);
#12034=ORIENTED_EDGE('',*,*,#8935,.T.);
#12035=ORIENTED_EDGE('',*,*,#8935,.F.);
#12036=ORIENTED_EDGE('',*,*,#8905,.F.);
#12037=ORIENTED_EDGE('',*,*,#8881,.F.);
#12038=ORIENTED_EDGE('',*,*,#8907,.F.);
#12039=ORIENTED_EDGE('',*,*,#8934,.F.);
#12040=ORIENTED_EDGE('',*,*,#8931,.F.);
#12041=ORIENTED_EDGE('',*,*,#8933,.F.);
#12042=ORIENTED_EDGE('',*,*,#8900,.T.);
#12043=ORIENTED_EDGE('',*,*,#8928,.F.);
#12044=ORIENTED_EDGE('',*,*,#8902,.T.);
#12045=ORIENTED_EDGE('',*,*,#8932,.F.);
#12046=ORIENTED_EDGE('',*,*,#8879,.F.);
#12047=ORIENTED_EDGE('',*,*,#8909,.F.);
#12048=ORIENTED_EDGE('',*,*,#8930,.F.);
#12049=ORIENTED_EDGE('',*,*,#8926,.F.);
#12050=ORIENTED_EDGE('',*,*,#8929,.F.);
#12051=ORIENTED_EDGE('',*,*,#8898,.T.);
#12052=ORIENTED_EDGE('',*,*,#8923,.F.);
#12053=ORIENTED_EDGE('',*,*,#8911,.F.);
#12054=ORIENTED_EDGE('',*,*,#8925,.F.);
#12055=ORIENTED_EDGE('',*,*,#8921,.F.);
#12056=ORIENTED_EDGE('',*,*,#8924,.F.);
#12057=ORIENTED_EDGE('',*,*,#8896,.T.);
#12058=ORIENTED_EDGE('',*,*,#8918,.F.);
#12059=ORIENTED_EDGE('',*,*,#8913,.F.);
#12060=ORIENTED_EDGE('',*,*,#8920,.F.);
#12061=ORIENTED_EDGE('',*,*,#8889,.F.);
#12062=ORIENTED_EDGE('',*,*,#8919,.F.);
#12063=ORIENTED_EDGE('',*,*,#8894,.T.);
#12064=ORIENTED_EDGE('',*,*,#8891,.F.);
#12065=ORIENTED_EDGE('',*,*,#8914,.F.);
#12066=ORIENTED_EDGE('',*,*,#8887,.F.);
#12067=ORIENTED_EDGE('',*,*,#8883,.F.);
#12068=ORIENTED_EDGE('',*,*,#8893,.T.);
#12069=ORIENTED_EDGE('',*,*,#8868,.T.);
#12070=ORIENTED_EDGE('',*,*,#8885,.F.);
#12071=ORIENTED_EDGE('',*,*,#8858,.F.);
#12072=ORIENTED_EDGE('',*,*,#8904,.T.);
#12073=ORIENTED_EDGE('',*,*,#8836,.T.);
#12074=ORIENTED_EDGE('',*,*,#8936,.T.);
#12075=ORIENTED_EDGE('',*,*,#8834,.T.);
#12076=ORIENTED_EDGE('',*,*,#8831,.T.);
#12077=ORIENTED_EDGE('',*,*,#8828,.T.);
#12078=ORIENTED_EDGE('',*,*,#8825,.T.);
#12079=ORIENTED_EDGE('',*,*,#8915,.T.);
#12080=ORIENTED_EDGE('',*,*,#8843,.F.);
#12081=ORIENTED_EDGE('',*,*,#8847,.F.);
#12082=ORIENTED_EDGE('',*,*,#8850,.F.);
#12083=ORIENTED_EDGE('',*,*,#8853,.F.);
#12084=ORIENTED_EDGE('',*,*,#8873,.F.);
#12085=ORIENTED_EDGE('',*,*,#8835,.T.);
#12086=ORIENTED_EDGE('',*,*,#8937,.T.);
#12087=ORIENTED_EDGE('',*,*,#8832,.F.);
#12088=ORIENTED_EDGE('',*,*,#8936,.F.);
#12089=ORIENTED_EDGE('',*,*,#8838,.F.);
#12090=ORIENTED_EDGE('',*,*,#8903,.T.);
#12091=ORIENTED_EDGE('',*,*,#8856,.T.);
#12092=ORIENTED_EDGE('',*,*,#8874,.T.);
#12093=ORIENTED_EDGE('',*,*,#8854,.T.);
#12094=ORIENTED_EDGE('',*,*,#8851,.T.);
#12095=ORIENTED_EDGE('',*,*,#8848,.T.);
#12096=ORIENTED_EDGE('',*,*,#8845,.T.);
#12097=ORIENTED_EDGE('',*,*,#8841,.T.);
#12098=ORIENTED_EDGE('',*,*,#8916,.T.);
#12099=ORIENTED_EDGE('',*,*,#8823,.F.);
#12100=ORIENTED_EDGE('',*,*,#8827,.F.);
#12101=ORIENTED_EDGE('',*,*,#8830,.F.);
#12102=ORIENTED_EDGE('',*,*,#8833,.F.);
#12103=ORIENTED_EDGE('',*,*,#8937,.F.);
#12104=ORIENTED_EDGE('',*,*,#8877,.F.);
#12105=ORIENTED_EDGE('',*,*,#8886,.F.);
#12106=ORIENTED_EDGE('',*,*,#8866,.T.);
#12107=ORIENTED_EDGE('',*,*,#8872,.T.);
#12108=ORIENTED_EDGE('',*,*,#8861,.T.);
#14255=PLANE('',#16482);
#14256=PLANE('',#16484);
#14257=PLANE('',#16486);
#14258=PLANE('',#16493);
#14259=PLANE('',#16500);
#14260=PLANE('',#16501);
#14261=PLANE('',#16502);
#14262=PLANE('',#16503);
#14263=PLANE('',#16518);
#15053=ADVANCED_FACE('',(#2085),#1233,.F.);
#15054=ADVANCED_FACE('',(#2086),#1234,.F.);
#15055=ADVANCED_FACE('',(#2087),#1235,.F.);
#15056=ADVANCED_FACE('',(#2088),#1236,.F.);
#15057=ADVANCED_FACE('',(#2089),#1237,.F.);
#15058=ADVANCED_FACE('',(#2090),#1238,.F.);
#15059=ADVANCED_FACE('',(#2091),#1239,.F.);
#15060=ADVANCED_FACE('',(#2092),#1240,.F.);
#15061=ADVANCED_FACE('',(#2093),#1241,.F.);
#15062=ADVANCED_FACE('',(#2094),#1242,.F.);
#15063=ADVANCED_FACE('',(#2095),#1243,.F.);
#15064=ADVANCED_FACE('',(#2096),#603,.T.);
#15065=ADVANCED_FACE('',(#2097),#1244,.T.);
#15066=ADVANCED_FACE('',(#2098),#604,.T.);
#15067=ADVANCED_FACE('',(#2099),#1245,.F.);
#15068=ADVANCED_FACE('',(#2100),#605,.T.);
#15069=ADVANCED_FACE('',(#2101),#14255,.F.);
#15070=ADVANCED_FACE('',(#2102),#14256,.F.);
#15071=ADVANCED_FACE('',(#2103,#1601),#14257,.T.);
#15072=ADVANCED_FACE('',(#2104,#1602),#14258,.F.);
#15073=ADVANCED_FACE('',(#2105),#14259,.F.);
#15074=ADVANCED_FACE('',(#2106),#14260,.F.);
#15075=ADVANCED_FACE('',(#2107),#14261,.F.);
#15076=ADVANCED_FACE('',(#2108),#14262,.F.);
#15077=ADVANCED_FACE('',(#2109),#606,.T.);
#15078=ADVANCED_FACE('',(#2110),#607,.T.);
#15079=ADVANCED_FACE('',(#2111),#608,.T.);
#15080=ADVANCED_FACE('',(#2112),#609,.T.);
#15081=ADVANCED_FACE('',(#2113),#610,.T.);
#15082=ADVANCED_FACE('',(#2114),#611,.T.);
#15083=ADVANCED_FACE('',(#2115),#612,.T.);
#15084=ADVANCED_FACE('',(#2116),#613,.T.);
#15085=ADVANCED_FACE('',(#2117),#614,.T.);
#15086=ADVANCED_FACE('',(#2118),#615,.T.);
#15087=ADVANCED_FACE('',(#2119),#616,.T.);
#15088=ADVANCED_FACE('',(#2120),#617,.T.);
#15089=ADVANCED_FACE('',(#2121),#315,.F.);
#15090=ADVANCED_FACE('',(#2122),#1246,.F.);
#15091=ADVANCED_FACE('',(#2123),#316,.F.);
#15092=ADVANCED_FACE('',(#2124),#1247,.T.);
#15093=ADVANCED_FACE('',(#2125),#14263,.T.);
#15571=CLOSED_SHELL('',(#15053,#15054,#15055,#15056,#15057,#15058,#15059,
#15060,#15061,#15062,#15063,#15064,#15065,#15066,#15067,#15068,#15069,#15070,
#15071,#15072,#15073,#15074,#15075,#15076,#15077,#15078,#15079,#15080,#15081,
#15082,#15083,#15084,#15085,#15086,#15087,#15088,#15089,#15090,#15091,#15092,
#15093));
#16451=AXIS2_PLACEMENT_3D('',#29139,#19048,#19049);
#16452=AXIS2_PLACEMENT_3D('',#29140,#19050,#19051);
#16453=AXIS2_PLACEMENT_3D('',#29161,#19053,#19054);
#16454=AXIS2_PLACEMENT_3D('',#29183,#19055,#19056);
#16455=AXIS2_PLACEMENT_3D('',#29229,#19058,#19059);
#16456=AXIS2_PLACEMENT_3D('',#29275,#19061,#19062);
#16457=AXIS2_PLACEMENT_3D('',#29321,#19064,#19065);
#16458=AXIS2_PLACEMENT_3D('',#29342,#19067,#19068);
#16459=AXIS2_PLACEMENT_3D('',#29362,#19069,#19070);
#16460=AXIS2_PLACEMENT_3D('',#29367,#19072,#19073);
#16461=AXIS2_PLACEMENT_3D('',#29376,#19074,#19075);
#16462=AXIS2_PLACEMENT_3D('',#29417,#19077,#19078);
#16463=AXIS2_PLACEMENT_3D('',#29454,#19079,#19080);
#16464=AXIS2_PLACEMENT_3D('',#29530,#19082,#19083);
#16465=AXIS2_PLACEMENT_3D('',#29606,#19085,#19086);
#16466=AXIS2_PLACEMENT_3D('',#29682,#19088,#19089);
#16467=AXIS2_PLACEMENT_3D('',#29706,#19091,#19092);
#16468=AXIS2_PLACEMENT_3D('',#29729,#19093,#19094);
#16469=AXIS2_PLACEMENT_3D('',#29731,#19095,#19096);
#16470=AXIS2_PLACEMENT_3D('',#29734,#19098,#19099);
#16471=AXIS2_PLACEMENT_3D('',#29735,#19100,#19101);
#16472=AXIS2_PLACEMENT_3D('',#29738,#19102,#19103);
#16473=AXIS2_PLACEMENT_3D('',#29740,#19105,#19106);
#16474=AXIS2_PLACEMENT_3D('',#29741,#19107,#19108);
#16475=AXIS2_PLACEMENT_3D('',#29745,#19110,#19111);
#16476=AXIS2_PLACEMENT_3D('',#29747,#19112,#19113);
#16477=AXIS2_PLACEMENT_3D('',#29769,#19114,#19115);
#16478=AXIS2_PLACEMENT_3D('',#29770,#19116,#19117);
#16479=AXIS2_PLACEMENT_3D('',#29771,#19118,#19119);
#16480=AXIS2_PLACEMENT_3D('',#29844,#19120,#19121);
#16481=AXIS2_PLACEMENT_3D('',#29849,#19122,#19123);
#16482=AXIS2_PLACEMENT_3D('',#29850,#19124,#19125);
#16483=AXIS2_PLACEMENT_3D('',#29852,#19126,#19127);
#16484=AXIS2_PLACEMENT_3D('',#29872,#19132,#19133);
#16485=AXIS2_PLACEMENT_3D('',#29878,#19134,#19135);
#16486=AXIS2_PLACEMENT_3D('',#29896,#19139,#19140);
#16487=AXIS2_PLACEMENT_3D('',#29897,#19141,#19142);
#16488=AXIS2_PLACEMENT_3D('',#29899,#19143,#19144);
#16489=AXIS2_PLACEMENT_3D('',#29903,#19146,#19147);
#16490=AXIS2_PLACEMENT_3D('',#29907,#19149,#19150);
#16491=AXIS2_PLACEMENT_3D('',#29911,#19152,#19153);
#16492=AXIS2_PLACEMENT_3D('',#29914,#19155,#19156);
#16493=AXIS2_PLACEMENT_3D('',#29951,#19157,#19158);
#16494=AXIS2_PLACEMENT_3D('',#29953,#19159,#19160);
#16495=AXIS2_PLACEMENT_3D('',#29957,#19162,#19163);
#16496=AXIS2_PLACEMENT_3D('',#29961,#19165,#19166);
#16497=AXIS2_PLACEMENT_3D('',#29965,#19168,#19169);
#16498=AXIS2_PLACEMENT_3D('',#29968,#19171,#19172);
#16499=AXIS2_PLACEMENT_3D('',#29969,#19173,#19174);
#16500=AXIS2_PLACEMENT_3D('',#30004,#19175,#19176);
#16501=AXIS2_PLACEMENT_3D('',#30020,#19178,#19179);
#16502=AXIS2_PLACEMENT_3D('',#30036,#19181,#19182);
#16503=AXIS2_PLACEMENT_3D('',#30052,#19184,#19185);
#16504=AXIS2_PLACEMENT_3D('',#30065,#19186,#19187);
#16505=AXIS2_PLACEMENT_3D('',#30066,#19188,#19189);
#16506=AXIS2_PLACEMENT_3D('',#30067,#19190,#19191);
#16507=AXIS2_PLACEMENT_3D('',#30068,#19192,#19193);
#16508=AXIS2_PLACEMENT_3D('',#30069,#19194,#19195);
#16509=AXIS2_PLACEMENT_3D('',#30070,#19196,#19197);
#16510=AXIS2_PLACEMENT_3D('',#30071,#19198,#19199);
#16511=AXIS2_PLACEMENT_3D('',#30072,#19200,#19201);
#16512=AXIS2_PLACEMENT_3D('',#30073,#19202,#19203);
#16513=AXIS2_PLACEMENT_3D('',#30074,#19204,#19205);
#16514=AXIS2_PLACEMENT_3D('',#30075,#19206,#19207);
#16515=AXIS2_PLACEMENT_3D('',#30076,#19208,#19209);
#16516=AXIS2_PLACEMENT_3D('',#30372,#19210,#19211);
#16517=AXIS2_PLACEMENT_3D('',#30668,#19212,#19213);
#16518=AXIS2_PLACEMENT_3D('',#30669,#19214,#19215);
#19048=DIRECTION('axis',(0.,0.,1.));
#19049=DIRECTION('refdir',(1.,0.,0.));
#19050=DIRECTION('center_axis',(-7.2837465494537E-29,-1.,-1.47831161133771E-14));
#19051=DIRECTION('ref_axis',(-1.,0.,4.92707118958683E-15));
#19052=DIRECTION('',(-7.2837465494537E-29,-1.,-1.47831161133771E-14));
#19053=DIRECTION('center_axis',(6.93889390390723E-18,-1.,-7.50998708063543E-18));
#19054=DIRECTION('ref_axis',(-1.,0.,4.92707118958683E-15));
#19055=DIRECTION('center_axis',(-7.2837465494537E-29,-1.,-1.47831161133771E-14));
#19056=DIRECTION('ref_axis',(-1.,0.,4.92707118958683E-15));
#19057=DIRECTION('',(-7.2837465494537E-29,-1.,-1.47831161133771E-14));
#19058=DIRECTION('center_axis',(-7.2837465494537E-29,-1.,-1.47831161133771E-14));
#19059=DIRECTION('ref_axis',(-1.,0.,4.92707118958683E-15));
#19060=DIRECTION('',(-7.2837465494537E-29,-1.,-1.47831161133771E-14));
#19061=DIRECTION('center_axis',(-7.2837465494537E-29,-1.,-1.47831161133771E-14));
#19062=DIRECTION('ref_axis',(-1.,0.,4.92707118958683E-15));
#19063=DIRECTION('',(-7.2837465494537E-29,-1.,-1.47831161133771E-14));
#19064=DIRECTION('center_axis',(-7.2837465494537E-29,-1.,-1.47831161133771E-14));
#19065=DIRECTION('ref_axis',(-1.,0.,4.92707118958683E-15));
#19066=DIRECTION('',(-7.2837465494537E-29,-1.,-1.47831161133771E-14));
#19067=DIRECTION('center_axis',(-6.93889390390723E-18,1.,7.50998708063543E-18));
#19068=DIRECTION('ref_axis',(-1.,0.,4.92707118958683E-15));
#19069=DIRECTION('center_axis',(6.93889390390723E-18,-1.,7.50998708063543E-18));
#19070=DIRECTION('ref_axis',(3.2531186322964E-16,-7.50998708063542E-18,
-1.));
#19071=DIRECTION('',(6.93889390390723E-18,-1.,7.50998708063542E-18));
#19072=DIRECTION('center_axis',(-6.93889390390723E-18,1.,-7.50998708063543E-18));
#19073=DIRECTION('ref_axis',(-3.2531186322964E-16,7.50998708063542E-18,
1.));
#19074=DIRECTION('center_axis',(6.93889390390723E-18,-1.,7.50998708063543E-18));
#19075=DIRECTION('ref_axis',(3.2531186322964E-16,-7.50998708063542E-18,
-1.));
#19076=DIRECTION('',(6.93889390390723E-18,-1.,7.50998708063542E-18));
#19077=DIRECTION('center_axis',(-6.93889390390723E-18,1.,-7.50998708063543E-18));
#19078=DIRECTION('ref_axis',(-3.2531186322964E-16,7.50998708063542E-18,
1.));
#19079=DIRECTION('center_axis',(6.93889390390723E-18,-1.,7.50998708063543E-18));
#19080=DIRECTION('ref_axis',(3.2531186322964E-16,-7.50998708063542E-18,
-1.));
#19081=DIRECTION('',(6.93889390390723E-18,-1.,7.50998708063542E-18));
#19082=DIRECTION('center_axis',(6.93889390390723E-18,-1.,7.50998708063543E-18));
#19083=DIRECTION('ref_axis',(3.2531186322964E-16,-7.50998708063542E-18,
-1.));
#19084=DIRECTION('',(6.93889390390723E-18,-1.,7.50998708063542E-18));
#19085=DIRECTION('center_axis',(6.93889390390723E-18,-1.,7.50998708063543E-18));
#19086=DIRECTION('ref_axis',(3.2531186322964E-16,-7.50998708063542E-18,
-1.));
#19087=DIRECTION('',(6.93889390390723E-18,-1.,7.50998708063542E-18));
#19088=DIRECTION('center_axis',(6.93889390390723E-18,-1.,7.50998708063543E-18));
#19089=DIRECTION('ref_axis',(3.2531186322964E-16,-7.50998708063542E-18,
-1.));
#19090=DIRECTION('',(6.93889390390723E-18,-1.,7.50998708063542E-18));
#19091=DIRECTION('center_axis',(-6.93889390390723E-18,1.,-7.50998708063543E-18));
#19092=DIRECTION('ref_axis',(-3.2531186322964E-16,7.50998708063542E-18,
1.));
#19093=DIRECTION('center_axis',(-0.866025403784438,-0.500000000000002,2.85483331249634E-16));
#19094=DIRECTION('ref_axis',(0.500000000000002,-0.866025403784438,-1.56152092020898E-16));
#19095=DIRECTION('center_axis',(-0.866025403784438,-0.500000000000002,2.85483331249634E-16));
#19096=DIRECTION('ref_axis',(-0.500000000000002,0.866025403784438,-2.11601299807821E-14));
#19097=DIRECTION('',(0.96592582628907,-0.258819045102516,-2.25687796983236E-16));
#19098=DIRECTION('center_axis',(0.866025403784438,0.500000000000001,-2.85483331249634E-16));
#19099=DIRECTION('ref_axis',(-0.500000000000001,0.866025403784438,1.56152092020898E-16));
#19100=DIRECTION('center_axis',(-0.866025403784438,-0.500000000000001,2.85483331249634E-16));
#19101=DIRECTION('ref_axis',(0.500000000000001,-0.866025403784438,-1.56152092020897E-16));
#19102=DIRECTION('center_axis',(0.866025403784438,0.500000000000001,-2.85483331249634E-16));
#19103=DIRECTION('ref_axis',(-0.500000000000001,0.866025403784438,1.56152092020897E-16));
#19104=DIRECTION('',(0.866025403784438,0.500000000000001,-2.85483331249634E-16));
#19105=DIRECTION('center_axis',(0.866025403784438,0.500000000000001,-2.85483331249634E-16));
#19106=DIRECTION('ref_axis',(-0.500000000000001,0.866025403784438,1.56152092020897E-16));
#19107=DIRECTION('center_axis',(0.866025403784438,0.500000000000001,-2.85483331249634E-16));
#19108=DIRECTION('ref_axis',(-0.500000000000001,0.866025403784438,1.56152092020897E-16));
#19109=DIRECTION('',(-0.965925826289068,0.258819045102522,3.98879008230333E-16));
#19110=DIRECTION('center_axis',(-0.866025403784438,-0.500000000000001,2.85483331249634E-16));
#19111=DIRECTION('ref_axis',(0.500000000000001,-0.866025403784438,-1.56152092020896E-16));
#19112=DIRECTION('center_axis',(-0.866025403784166,-1.15935552460568E-13,
0.500000000000473));
#19113=DIRECTION('ref_axis',(-0.327326835368636,-0.75592894599349,-0.56694670953867));
#19114=DIRECTION('center_axis',(-0.86602540378437,-3.08582405011455E-14,
-0.500000000000119));
#19115=DIRECTION('ref_axis',(0.327326835357387,0.75592894601267,-0.566946709519592));
#19116=DIRECTION('center_axis',(-0.866025403784438,-0.500000000000001,2.85483331249634E-16));
#19117=DIRECTION('ref_axis',(0.500000000000001,-0.866025403784438,-1.56152092020896E-16));
#19118=DIRECTION('center_axis',(6.93889390390723E-18,-1.,7.50998708063543E-18));
#19119=DIRECTION('ref_axis',(3.2531186322964E-16,-7.50998708063542E-18,
-1.));
#19120=DIRECTION('center_axis',(6.93889390390723E-18,-1.,7.50998708063543E-18));
#19121=DIRECTION('ref_axis',(3.2531186322964E-16,-7.50998708063542E-18,
-1.));
#19122=DIRECTION('center_axis',(6.93889390390723E-18,-1.,7.50998708063543E-18));
#19123=DIRECTION('ref_axis',(3.2531186322964E-16,-7.50998708063542E-18,
-1.));
#19124=DIRECTION('center_axis',(-0.866025403784439,3.46944695195362E-18,
-0.5));
#19125=DIRECTION('ref_axis',(-0.5,-3.46944695195356E-18,0.866025403784439));
#19126=DIRECTION('center_axis',(-0.86602540378444,3.39006491526626E-15,
-0.499999999999998));
#19127=DIRECTION('ref_axis',(0.327326835353988,0.755928946018457,-0.566946709513838));
#19128=DIRECTION('',(0.5,1.73472347597681E-18,-0.866025403784439));
#19129=DIRECTION('',(6.93889390390723E-18,-1.,7.50998708063543E-18));
#19130=DIRECTION('',(0.5,1.73472347597681E-18,-0.866025403784439));
#19131=DIRECTION('',(6.93889390390723E-18,-1.,7.50998708063543E-18));
#19132=DIRECTION('center_axis',(-0.866025403784438,-1.73472347597681E-18,
0.5));
#19133=DIRECTION('ref_axis',(0.5,-8.67361737988409E-18,0.866025403784438));
#19134=DIRECTION('center_axis',(-0.866025403784443,6.78860499282057E-15,
0.499999999999992));
#19135=DIRECTION('ref_axis',(-0.327326835353985,-0.755928946018458,-0.566946709513837));
#19136=DIRECTION('',(-0.5,1.04083408558608E-17,-0.866025403784438));
#19137=DIRECTION('',(6.93889390390723E-18,-1.,7.50998708063543E-18));
#19138=DIRECTION('',(-0.5,1.04083408558608E-17,-0.866025403784438));
#19139=DIRECTION('center_axis',(-6.93889390390723E-18,1.,7.50998708063543E-18));
#19140=DIRECTION('ref_axis',(-3.2531186322964E-16,-7.50998708063543E-18,
1.));
#19141=DIRECTION('center_axis',(6.93889390390723E-18,-1.,7.50998708063543E-18));
#19142=DIRECTION('ref_axis',(3.2531186322964E-16,-7.50998708063542E-18,
-1.));
#19143=DIRECTION('center_axis',(6.93889390390723E-18,-1.,7.50998708063543E-18));
#19144=DIRECTION('ref_axis',(3.2531186322964E-16,-7.50998708063542E-18,
-1.));
#19145=DIRECTION('',(-1.,6.93889390390723E-18,3.2531186322964E-16));
#19146=DIRECTION('center_axis',(6.93889390390723E-18,-1.,7.50998708063543E-18));
#19147=DIRECTION('ref_axis',(3.2531186322964E-16,-7.50998708063542E-18,
-1.));
#19148=DIRECTION('',(-0.5,-3.46944695195356E-18,0.866025403784438));
#19149=DIRECTION('center_axis',(6.93889390390723E-18,-1.,7.50998708063543E-18));
#19150=DIRECTION('ref_axis',(3.2531186322964E-16,-7.50998708063542E-18,
-1.));
#19151=DIRECTION('',(0.5,-8.67361737988404E-18,0.866025403784438));
#19152=DIRECTION('center_axis',(6.93889390390723E-18,-1.,7.50998708063543E-18));
#19153=DIRECTION('ref_axis',(3.2531186322964E-16,-7.50998708063542E-18,
-1.));
#19154=DIRECTION('',(1.,-6.93889390390723E-18,-3.2531186322964E-16));
#19155=DIRECTION('center_axis',(6.93889390390723E-18,-1.,7.50998708063543E-18));
#19156=DIRECTION('ref_axis',(3.2531186322964E-16,-7.50998708063542E-18,
-1.));
#19157=DIRECTION('center_axis',(-6.93889390390723E-18,1.,7.50998708063543E-18));
#19158=DIRECTION('ref_axis',(-3.2531186322964E-16,-7.50998708063543E-18,
1.));
#19159=DIRECTION('center_axis',(6.93889390390723E-18,-1.,7.50998708063543E-18));
#19160=DIRECTION('ref_axis',(3.2531186322964E-16,-7.50998708063542E-18,
-1.));
#19161=DIRECTION('',(1.,-6.93889390390723E-18,-3.2531186322964E-16));
#19162=DIRECTION('center_axis',(6.93889390390723E-18,-1.,7.50998708063543E-18));
#19163=DIRECTION('ref_axis',(3.2531186322964E-16,-7.50998708063542E-18,
-1.));
#19164=DIRECTION('',(0.5,-8.67361737988404E-18,0.866025403784438));
#19165=DIRECTION('center_axis',(6.93889390390723E-18,-1.,7.50998708063543E-18));
#19166=DIRECTION('ref_axis',(3.2531186322964E-16,-7.50998708063542E-18,
-1.));
#19167=DIRECTION('',(-0.5,-3.46944695195356E-18,0.866025403784438));
#19168=DIRECTION('center_axis',(6.93889390390723E-18,-1.,7.50998708063543E-18));
#19169=DIRECTION('ref_axis',(3.2531186322964E-16,-7.50998708063542E-18,
-1.));
#19170=DIRECTION('',(-1.,6.93889390390723E-18,1.99119960773767E-16));
#19171=DIRECTION('center_axis',(6.93889390390723E-18,-1.,7.50998708063543E-18));
#19172=DIRECTION('ref_axis',(3.2531186322964E-16,-7.50998708063542E-18,
-1.));
#19173=DIRECTION('center_axis',(6.93889390390723E-18,-1.,7.50998708063543E-18));
#19174=DIRECTION('ref_axis',(3.2531186322964E-16,-7.50998708063542E-18,
-1.));
#19175=DIRECTION('center_axis',(1.99119960773767E-16,-7.50998708063543E-18,
1.));
#19176=DIRECTION('ref_axis',(1.,-6.93889390390723E-18,-1.99119960773767E-16));
#19177=DIRECTION('',(6.93889390390723E-18,-1.,7.50998708063543E-18));
#19178=DIRECTION('center_axis',(0.866025403784438,-6.93889390390723E-18,
0.5));
#19179=DIRECTION('ref_axis',(0.5,3.46944695195361E-18,-0.866025403784438));
#19180=DIRECTION('',(6.93889390390723E-18,-1.,7.50998708063543E-18));
#19181=DIRECTION('center_axis',(0.866025403784439,3.46944695195364E-18,
-0.5));
#19182=DIRECTION('ref_axis',(-0.5,1.04083408558609E-17,-0.866025403784439));
#19183=DIRECTION('',(6.93889390390723E-18,-1.,7.50998708063543E-18));
#19184=DIRECTION('center_axis',(-3.2531186322964E-16,7.50998708063543E-18,
-1.));
#19185=DIRECTION('ref_axis',(-1.,6.93889390390723E-18,3.2531186322964E-16));
#19186=DIRECTION('center_axis',(-6.93889390390723E-18,1.,-7.50998708063543E-18));
#19187=DIRECTION('ref_axis',(-3.2531186322964E-16,7.50998708063542E-18,
1.));
#19188=DIRECTION('center_axis',(-6.93889390390723E-18,1.,-7.50998708063543E-18));
#19189=DIRECTION('ref_axis',(-3.2531186322964E-16,7.50998708063542E-18,
1.));
#19190=DIRECTION('center_axis',(6.93889390390723E-18,-1.,7.50998708063543E-18));
#19191=DIRECTION('ref_axis',(3.2531186322964E-16,-7.50998708063542E-18,
-1.));
#19192=DIRECTION('center_axis',(6.93889390390723E-18,-1.,7.50998708063543E-18));
#19193=DIRECTION('ref_axis',(3.2531186322964E-16,-7.50998708063542E-18,
-1.));
#19194=DIRECTION('center_axis',(-6.93889390390723E-18,1.,-7.50998708063543E-18));
#19195=DIRECTION('ref_axis',(-3.2531186322964E-16,7.50998708063542E-18,
1.));
#19196=DIRECTION('center_axis',(6.93889390390723E-18,-1.,7.50998708063543E-18));
#19197=DIRECTION('ref_axis',(3.2531186322964E-16,-7.50998708063542E-18,
-1.));
#19198=DIRECTION('center_axis',(-6.93889390390723E-18,1.,-7.50998708063543E-18));
#19199=DIRECTION('ref_axis',(-3.2531186322964E-16,7.50998708063542E-18,
1.));
#19200=DIRECTION('center_axis',(6.93889390390723E-18,-1.,7.50998708063543E-18));
#19201=DIRECTION('ref_axis',(3.2531186322964E-16,-7.50998708063542E-18,
-1.));
#19202=DIRECTION('center_axis',(-6.93889390390723E-18,1.,-7.50998708063543E-18));
#19203=DIRECTION('ref_axis',(-3.2531186322964E-16,7.50998708063542E-18,
1.));
#19204=DIRECTION('center_axis',(6.93889390390723E-18,-1.,7.50998708063543E-18));
#19205=DIRECTION('ref_axis',(3.2531186322964E-16,-7.50998708063542E-18,
-1.));
#19206=DIRECTION('center_axis',(-6.93889390390723E-18,1.,-7.50998708063543E-18));
#19207=DIRECTION('ref_axis',(-3.2531186322964E-16,7.50998708063542E-18,
1.));
#19208=DIRECTION('center_axis',(6.93889390390723E-18,-1.,7.50998708063543E-18));
#19209=DIRECTION('ref_axis',(3.2531186322964E-16,-7.50998708063542E-18,
-1.));
#19210=DIRECTION('center_axis',(-7.2837465494537E-29,-1.,-1.47831161133771E-14));
#19211=DIRECTION('ref_axis',(-1.,0.,4.92707118958683E-15));
#19212=DIRECTION('center_axis',(0.866025403784438,0.500000000000001,-2.85483331249634E-16));
#19213=DIRECTION('ref_axis',(0.500000000000001,-0.866025403784438,4.40720468639446E-15));
#19214=DIRECTION('center_axis',(0.866025403784438,0.500000000000001,-2.85483331249634E-16));
#19215=DIRECTION('ref_axis',(-0.500000000000001,0.866025403784438,1.56152092020897E-16));
#29139=CARTESIAN_POINT('',(0.,0.,0.));
#29140=CARTESIAN_POINT('Origin',(-3.44169137633799E-14,15.9887500034686,
-8.78459658321108E-14));
#29141=CARTESIAN_POINT('',(6.56268467749993,2.3362500034686,-1.60601788046217E-13));
#29142=CARTESIAN_POINT('',(6.56268467750004,1.7012500034686,-1.65295427412214E-13));
#29143=CARTESIAN_POINT('',(6.56268467749992,15.9887500034686,-1.19377083354552E-13));
#29144=CARTESIAN_POINT('',(-3.17934379362961,0.,-5.74113257277709));
#29145=CARTESIAN_POINT('Ctrl Pts',(6.56268467750004,1.7012500034686,0.));
#29146=CARTESIAN_POINT('Ctrl Pts',(6.56268467750014,1.57425000346862,2.13234551188562));
#29147=CARTESIAN_POINT('Ctrl Pts',(5.30932343282148,1.44725000346863,3.85744926888032));
#29148=CARTESIAN_POINT('Ctrl Pts',(4.05596218814318,1.32025000346859,5.58255302587488));
#29149=CARTESIAN_POINT('Ctrl Pts',(2.0279810940716,1.19325000346859,6.2414840269267));
#29150=CARTESIAN_POINT('Ctrl Pts',(0.,1.06625000346873,6.90041502797853));
#29151=CARTESIAN_POINT('Ctrl Pts',(-2.0279810940716,0.939250003468617,6.2414840269267));
#29152=CARTESIAN_POINT('Ctrl Pts',(-4.05596218814312,0.81225000346864,5.58255302587488));
#29153=CARTESIAN_POINT('Ctrl Pts',(-5.30932343282148,0.685250003468529,
3.85744926888032));
#29154=CARTESIAN_POINT('Ctrl Pts',(-6.56268467749997,0.558250003468608,
2.13234551188562));
#29155=CARTESIAN_POINT('Ctrl Pts',(-6.5626846775001,0.431250003468608,0.));
#29156=CARTESIAN_POINT('Ctrl Pts',(-6.56268467750003,0.304250003468635,
-2.13234551188562));
#29157=CARTESIAN_POINT('Ctrl Pts',(-5.30932343282153,0.177250003468632,
-3.85744926888032));
#29158=CARTESIAN_POINT('Ctrl Pts',(-4.45333360667123,0.0905146680793477,
-5.03561818970082));
#29159=CARTESIAN_POINT('Ctrl Pts',(-3.17934379362961,0.,-5.74113257277708));
#29160=CARTESIAN_POINT('',(5.75296004380515,0.,-3.15789184594317));
#29161=CARTESIAN_POINT('Origin',(-3.4416913763381E-14,0.,-3.24209513641145E-13));
#29162=CARTESIAN_POINT('Ctrl Pts',(6.56268467749993,2.3362500034686,0.));
#29163=CARTESIAN_POINT('Ctrl Pts',(6.56268467750003,2.20925000346864,2.13234551188562));
#29164=CARTESIAN_POINT('Ctrl Pts',(5.30932343282159,2.08225000346862,3.85744926888032));
#29165=CARTESIAN_POINT('Ctrl Pts',(4.05596218814324,1.95525000346861,5.58255302587488));
#29166=CARTESIAN_POINT('Ctrl Pts',(2.02798109407148,1.82825000346865,6.2414840269267));
#29167=CARTESIAN_POINT('Ctrl Pts',(1.1673575708729E-13,1.70125000346858,
6.90041502797853));
#29168=CARTESIAN_POINT('Ctrl Pts',(-2.02798109407148,1.57425000346872,6.2414840269267));
#29169=CARTESIAN_POINT('Ctrl Pts',(-4.05596218814306,1.44725000346872,5.58255302587488));
#29170=CARTESIAN_POINT('Ctrl Pts',(-5.30932343282159,1.32025000346858,3.85744926888032));
#29171=CARTESIAN_POINT('Ctrl Pts',(-6.56268467750003,1.19325000346869,2.13234551188562));
#29172=CARTESIAN_POINT('Ctrl Pts',(-6.56268467749999,1.06625000346861,0.));
#29173=CARTESIAN_POINT('Ctrl Pts',(-6.56268467749997,0.939250003468656,
-2.13234551188562));
#29174=CARTESIAN_POINT('Ctrl Pts',(-5.30932343282164,0.812250003468629,
-3.85744926888032));
#29175=CARTESIAN_POINT('Ctrl Pts',(-4.05596218814312,0.685250003468624,
-5.58255302587488));
#29176=CARTESIAN_POINT('Ctrl Pts',(-2.02798109407154,0.558250003468708,
-6.2414840269267));
#29177=CARTESIAN_POINT('Ctrl Pts',(0.,0.431250003468709,-6.90041502797853));
#29178=CARTESIAN_POINT('Ctrl Pts',(2.02798109407154,0.30425000346862,-6.2414840269267));
#29179=CARTESIAN_POINT('Ctrl Pts',(4.05596218814306,0.177250003468736,-5.58255302587488));
#29180=CARTESIAN_POINT('Ctrl Pts',(5.30932343282159,0.0502500034685882,
-3.85744926888032));
#29181=CARTESIAN_POINT('Ctrl Pts',(5.55326106788226,0.0255324052627934,
-3.52169791826031));
#29182=CARTESIAN_POINT('Ctrl Pts',(5.75296004380515,0.,-3.15789184594317));
#29183=CARTESIAN_POINT('Origin',(-3.44169137633799E-14,15.9887500034686,
-8.78459658321108E-14));
#29184=CARTESIAN_POINT('',(6.56268467749999,4.87625000346864,-1.41827230582227E-13));
#29185=CARTESIAN_POINT('',(6.5626846775001,4.24125000346864,-1.46520869948225E-13));
#29186=CARTESIAN_POINT('',(6.56268467749992,15.9887500034686,-1.19377083354552E-13));
#29187=CARTESIAN_POINT('Ctrl Pts',(6.5626846775001,4.24125000346864,0.));
#29188=CARTESIAN_POINT('Ctrl Pts',(6.56268467750003,4.1142500034687,2.13234551188562));
#29189=CARTESIAN_POINT('Ctrl Pts',(5.30932343282148,3.98725000346861,3.85744926888032));
#29190=CARTESIAN_POINT('Ctrl Pts',(4.05596218814318,3.86025000346873,5.58255302587488));
#29191=CARTESIAN_POINT('Ctrl Pts',(2.0279810940716,3.73325000346858,6.2414840269267));
#29192=CARTESIAN_POINT('Ctrl Pts',(0.,3.60625000346864,6.90041502797853));
#29193=CARTESIAN_POINT('Ctrl Pts',(-2.0279810940716,3.4792500034686,6.2414840269267));
#29194=CARTESIAN_POINT('Ctrl Pts',(-4.05596218814312,3.35225000346861,5.58255302587488));
#29195=CARTESIAN_POINT('Ctrl Pts',(-5.30932343282159,3.22525000346852,3.85744926888032));
#29196=CARTESIAN_POINT('Ctrl Pts',(-6.56268467749991,3.09825000346869,2.13234551188562));
#29197=CARTESIAN_POINT('Ctrl Pts',(-6.5626846775001,2.9712500034686,0.));
#29198=CARTESIAN_POINT('Ctrl Pts',(-6.56268467750003,2.8442500034686,-2.13234551188562));
#29199=CARTESIAN_POINT('Ctrl Pts',(-5.30932343282148,2.71725000346862,-3.85744926888032));
#29200=CARTESIAN_POINT('Ctrl Pts',(-4.05596218814306,2.59025000346863,-5.58255302587488));
#29201=CARTESIAN_POINT('Ctrl Pts',(-2.02798109407165,2.46325000346864,-6.2414840269267));
#29202=CARTESIAN_POINT('Ctrl Pts',(0.,2.3362500034686,-6.90041502797853));
#29203=CARTESIAN_POINT('Ctrl Pts',(2.02798109407165,2.20925000346861,-6.2414840269267));
#29204=CARTESIAN_POINT('Ctrl Pts',(4.05596218814312,2.08225000346851,-5.58255302587488));
#29205=CARTESIAN_POINT('Ctrl Pts',(5.30932343282148,1.95525000346858,-3.85744926888032));
#29206=CARTESIAN_POINT('Ctrl Pts',(6.56268467749997,1.82825000346865,-2.13234551188562));
#29207=CARTESIAN_POINT('Ctrl Pts',(6.56268467750004,1.7012500034686,0.));
#29208=CARTESIAN_POINT('Ctrl Pts',(6.56268467749999,4.87625000346864,0.));
#29209=CARTESIAN_POINT('Ctrl Pts',(6.56268467750008,4.74925000346872,2.13234551188562));
#29210=CARTESIAN_POINT('Ctrl Pts',(5.30932343282159,4.62225000346861,3.85744926888032));
#29211=CARTESIAN_POINT('Ctrl Pts',(4.05596218814312,4.49525000346869,5.58255302587488));
#29212=CARTESIAN_POINT('Ctrl Pts',(2.02798109407148,4.36825000346869,6.2414840269267));
#29213=CARTESIAN_POINT('Ctrl Pts',(0.,4.24125000346866,6.90041502797853));
#29214=CARTESIAN_POINT('Ctrl Pts',(-2.0279810940716,4.11425000346871,6.2414840269267));
#29215=CARTESIAN_POINT('Ctrl Pts',(-4.05596218814312,3.98725000346863,5.58255302587488));
#29216=CARTESIAN_POINT('Ctrl Pts',(-5.30932343282159,3.86025000346862,3.85744926888032));
#29217=CARTESIAN_POINT('Ctrl Pts',(-6.56268467749997,3.7332500034686,2.13234551188562));
#29218=CARTESIAN_POINT('Ctrl Pts',(-6.56268467749999,3.60625000346859,0.));
#29219=CARTESIAN_POINT('Ctrl Pts',(-6.56268467750008,3.47925000346862,-2.13234551188562));
#29220=CARTESIAN_POINT('Ctrl Pts',(-5.30932343282159,3.3522500034685,-3.85744926888032));
#29221=CARTESIAN_POINT('Ctrl Pts',(-4.05596218814312,3.22525000346859,-5.58255302587488));
#29222=CARTESIAN_POINT('Ctrl Pts',(-2.02798109407154,3.09825000346858,-6.2414840269267));
#29223=CARTESIAN_POINT('Ctrl Pts',(5.83678785436452E-14,2.97125000346862,
-6.90041502797853));
#29224=CARTESIAN_POINT('Ctrl Pts',(2.02798109407154,2.84425000346861,-6.2414840269267));
#29225=CARTESIAN_POINT('Ctrl Pts',(4.05596218814318,2.71725000346853,-5.58255302587488));
#29226=CARTESIAN_POINT('Ctrl Pts',(5.30932343282159,2.59025000346863,-3.85744926888032));
#29227=CARTESIAN_POINT('Ctrl Pts',(6.56268467750003,2.46325000346861,-2.13234551188562));
#29228=CARTESIAN_POINT('Ctrl Pts',(6.56268467749993,2.3362500034686,0.));
#29229=CARTESIAN_POINT('Origin',(-3.44169137633799E-14,15.9887500034686,
-8.78459658321108E-14));
#29230=CARTESIAN_POINT('',(6.56268467749999,7.41625000346852,-1.50808248733868E-13));
#29231=CARTESIAN_POINT('',(6.56268467749999,6.78125000346857,-1.55501888099865E-13));
#29232=CARTESIAN_POINT('',(6.56268467749992,15.9887500034686,-1.19377083354552E-13));
#29233=CARTESIAN_POINT('Ctrl Pts',(6.56268467749999,6.78125000346857,-5.55111512312578E-14));
#29234=CARTESIAN_POINT('Ctrl Pts',(6.56268467750003,6.65425000346861,2.13234551188562));
#29235=CARTESIAN_POINT('Ctrl Pts',(5.30932343282148,6.5272500034686,3.85744926888026));
#29236=CARTESIAN_POINT('Ctrl Pts',(4.05596218814318,6.40025000346864,5.58255302587488));
#29237=CARTESIAN_POINT('Ctrl Pts',(2.0279810940716,6.27325000346862,6.24148402692665));
#29238=CARTESIAN_POINT('Ctrl Pts',(-1.1673575708729E-13,6.14625000346872,
6.90041502797853));
#29239=CARTESIAN_POINT('Ctrl Pts',(-2.0279810940716,6.01925000346865,6.2414840269267));
#29240=CARTESIAN_POINT('Ctrl Pts',(-4.05596218814324,5.89225000346851,5.58255302587488));
#29241=CARTESIAN_POINT('Ctrl Pts',(-5.30932343282159,5.76525000346861,3.85744926888032));
#29242=CARTESIAN_POINT('Ctrl Pts',(-6.56268467750003,5.63825000346866,2.13234551188562));
#29243=CARTESIAN_POINT('Ctrl Pts',(-6.56268467750004,5.51125000346864,0.));
#29244=CARTESIAN_POINT('Ctrl Pts',(-6.56268467749997,5.38425000346863,-2.13234551188562));
#29245=CARTESIAN_POINT('Ctrl Pts',(-5.30932343282148,5.25725000346872,-3.85744926888032));
#29246=CARTESIAN_POINT('Ctrl Pts',(-4.05596218814318,5.13025000346865,-5.58255302587488));
#29247=CARTESIAN_POINT('Ctrl Pts',(-2.02798109407165,5.00325000346863,-6.2414840269267));
#29248=CARTESIAN_POINT('Ctrl Pts',(0.,4.87625000346868,-6.90041502797853));
#29249=CARTESIAN_POINT('Ctrl Pts',(2.02798109407154,4.7492500034686,-6.2414840269267));
#29250=CARTESIAN_POINT('Ctrl Pts',(4.05596218814312,4.62225000346859,-5.58255302587488));
#29251=CARTESIAN_POINT('Ctrl Pts',(5.30932343282148,4.49525000346862,-3.85744926888032));
#29252=CARTESIAN_POINT('Ctrl Pts',(6.56268467750008,4.36825000346862,-2.13234551188562));
#29253=CARTESIAN_POINT('Ctrl Pts',(6.5626846775001,4.24125000346864,0.));
#29254=CARTESIAN_POINT('Ctrl Pts',(6.56268467749999,7.41625000346852,-5.55111512312578E-14));
#29255=CARTESIAN_POINT('Ctrl Pts',(6.56268467749997,7.28925000346863,2.13234551188562));
#29256=CARTESIAN_POINT('Ctrl Pts',(5.30932343282159,7.1622500034686,3.85744926888026));
#29257=CARTESIAN_POINT('Ctrl Pts',(4.05596218814312,7.0352500034686,5.58255302587488));
#29258=CARTESIAN_POINT('Ctrl Pts',(2.02798109407154,6.90825000346851,6.24148402692665));
#29259=CARTESIAN_POINT('Ctrl Pts',(0.,6.78125000346874,6.90041502797853));
#29260=CARTESIAN_POINT('Ctrl Pts',(-2.0279810940716,6.65425000346853,6.24148402692665));
#29261=CARTESIAN_POINT('Ctrl Pts',(-4.05596218814312,6.52725000346859,5.58255302587488));
#29262=CARTESIAN_POINT('Ctrl Pts',(-5.30932343282159,6.40025000346872,3.85744926888026));
#29263=CARTESIAN_POINT('Ctrl Pts',(-6.56268467749997,6.27325000346868,2.13234551188562));
#29264=CARTESIAN_POINT('Ctrl Pts',(-6.56268467749993,6.14625000346863,0.));
#29265=CARTESIAN_POINT('Ctrl Pts',(-6.56268467749991,6.01925000346865,-2.13234551188562));
#29266=CARTESIAN_POINT('Ctrl Pts',(-5.30932343282159,5.8922500034686,-3.85744926888032));
#29267=CARTESIAN_POINT('Ctrl Pts',(-4.05596218814312,5.76525000346861,-5.58255302587488));
#29268=CARTESIAN_POINT('Ctrl Pts',(-2.02798109407154,5.63825000346863,-6.2414840269267));
#29269=CARTESIAN_POINT('Ctrl Pts',(0.,5.5112500034687,-6.90041502797853));
#29270=CARTESIAN_POINT('Ctrl Pts',(2.02798109407154,5.38425000346859,-6.2414840269267));
#29271=CARTESIAN_POINT('Ctrl Pts',(4.05596218814324,5.25725000346861,-5.58255302587488));
#29272=CARTESIAN_POINT('Ctrl Pts',(5.30932343282159,5.13025000346867,-3.85744926888032));
#29273=CARTESIAN_POINT('Ctrl Pts',(6.56268467750003,5.00325000346858,-2.13234551188562));
#29274=CARTESIAN_POINT('Ctrl Pts',(6.56268467749999,4.87625000346864,0.));
#29275=CARTESIAN_POINT('Origin',(-3.44169137633799E-14,15.9887500034686,
-8.78459658321108E-14));
#29276=CARTESIAN_POINT('',(6.56268467749999,9.95625000346861,-1.32033691269879E-13));
#29277=CARTESIAN_POINT('',(6.56268467749999,9.32125000346862,-1.36727330635876E-13));
#29278=CARTESIAN_POINT('',(6.56268467749992,15.9887500034686,-1.19377083354552E-13));
#29279=CARTESIAN_POINT('Ctrl Pts',(6.56268467749999,9.32125000346862,-5.55111512312578E-14));
#29280=CARTESIAN_POINT('Ctrl Pts',(6.56268467750003,9.19425000346858,2.13234551188562));
#29281=CARTESIAN_POINT('Ctrl Pts',(5.30932343282153,9.06725000346864,3.85744926888026));
#29282=CARTESIAN_POINT('Ctrl Pts',(4.05596218814318,8.94025000346872,5.58255302587488));
#29283=CARTESIAN_POINT('Ctrl Pts',(2.02798109407165,8.81325000346872,6.24148402692665));
#29284=CARTESIAN_POINT('Ctrl Pts',(1.1673575708729E-13,8.68625000346869,
6.90041502797853));
#29285=CARTESIAN_POINT('Ctrl Pts',(-2.0279810940716,8.55925000346869,6.24148402692665));
#29286=CARTESIAN_POINT('Ctrl Pts',(-4.05596218814306,8.4322500034686,5.58255302587488));
#29287=CARTESIAN_POINT('Ctrl Pts',(-5.30932343282159,8.3052500034686,3.85744926888026));
#29288=CARTESIAN_POINT('Ctrl Pts',(-6.56268467749991,8.17825000346862,2.13234551188562));
#29289=CARTESIAN_POINT('Ctrl Pts',(-6.56268467749999,8.05125000346868,-5.55111512312578E-14));
#29290=CARTESIAN_POINT('Ctrl Pts',(-6.56268467749997,7.92425000346871,-2.13234551188562));
#29291=CARTESIAN_POINT('Ctrl Pts',(-5.30932343282159,7.79725000346859,-3.85744926888038));
#29292=CARTESIAN_POINT('Ctrl Pts',(-4.05596218814306,7.67025000346873,-5.58255302587488));
#29293=CARTESIAN_POINT('Ctrl Pts',(-2.0279810940716,7.54325000346862,-6.24148402692676));
#29294=CARTESIAN_POINT('Ctrl Pts',(-1.1673575708729E-13,7.41625000346859,
-6.90041502797853));
#29295=CARTESIAN_POINT('Ctrl Pts',(2.02798109407154,7.28925000346869,-6.24148402692676));
#29296=CARTESIAN_POINT('Ctrl Pts',(4.05596218814318,7.16225000346861,-5.58255302587488));
#29297=CARTESIAN_POINT('Ctrl Pts',(5.30932343282153,7.03525000346861,-3.85744926888038));
#29298=CARTESIAN_POINT('Ctrl Pts',(6.56268467750008,6.90825000346864,-2.13234551188562));
#29299=CARTESIAN_POINT('Ctrl Pts',(6.56268467749999,6.78125000346857,-5.55111512312578E-14));
#29300=CARTESIAN_POINT('Ctrl Pts',(6.56268467749999,9.95625000346861,-5.55111512312578E-14));
#29301=CARTESIAN_POINT('Ctrl Pts',(6.56268467750008,9.8292500034686,2.13234551188562));
#29302=CARTESIAN_POINT('Ctrl Pts',(5.30932343282164,9.70225000346864,3.85744926888026));
#29303=CARTESIAN_POINT('Ctrl Pts',(4.05596218814312,9.57525000346868,5.58255302587488));
#29304=CARTESIAN_POINT('Ctrl Pts',(2.02798109407154,9.44825000346855,6.24148402692665));
#29305=CARTESIAN_POINT('Ctrl Pts',(0.,9.32125000346853,6.90041502797853));
#29306=CARTESIAN_POINT('Ctrl Pts',(-2.02798109407154,9.19425000346857,6.24148402692665));
#29307=CARTESIAN_POINT('Ctrl Pts',(-4.05596218814312,9.06725000346862,5.58255302587488));
#29308=CARTESIAN_POINT('Ctrl Pts',(-5.30932343282159,8.9402500034686,3.85744926888026));
#29309=CARTESIAN_POINT('Ctrl Pts',(-6.56268467749997,8.81325000346859,2.13234551188562));
#29310=CARTESIAN_POINT('Ctrl Pts',(-6.56268467749999,8.68625000346862,-5.55111512312578E-14));
#29311=CARTESIAN_POINT('Ctrl Pts',(-6.56268467750003,8.55925000346873,-2.13234551188562));
#29312=CARTESIAN_POINT('Ctrl Pts',(-5.30932343282159,8.43225000346859,-3.85744926888038));
#29313=CARTESIAN_POINT('Ctrl Pts',(-4.05596218814312,8.30525000346876,-5.58255302587488));
#29314=CARTESIAN_POINT('Ctrl Pts',(-2.02798109407148,8.17825000346861,-6.24148402692676));
#29315=CARTESIAN_POINT('Ctrl Pts',(0.,8.05125000346861,-6.90041502797853));
#29316=CARTESIAN_POINT('Ctrl Pts',(2.02798109407154,7.92425000346864,-6.24148402692676));
#29317=CARTESIAN_POINT('Ctrl Pts',(4.05596218814312,7.79725000346863,-5.58255302587488));
#29318=CARTESIAN_POINT('Ctrl Pts',(5.30932343282153,7.67025000346866,-3.85744926888038));
#29319=CARTESIAN_POINT('Ctrl Pts',(6.56268467750003,7.5432500034686,-2.13234551188562));
#29320=CARTESIAN_POINT('Ctrl Pts',(6.56268467749999,7.41625000346852,-5.55111512312578E-14));
#29321=CARTESIAN_POINT('Origin',(-3.44169137633799E-14,15.9887500034686,
-8.78459658321108E-14));
#29322=CARTESIAN_POINT('',(6.56268467749999,12.4962500034686,-1.1325913380589E-13));
#29323=CARTESIAN_POINT('',(6.56268467749999,11.8612500034686,-1.17952773171887E-13));
#29324=CARTESIAN_POINT('',(6.56268467749992,15.9887500034686,-1.19377083354552E-13));
#29325=CARTESIAN_POINT('',(-4.44227809454828,14.0999999999992,4.83063096365161));
#29326=CARTESIAN_POINT('Ctrl Pts',(-4.44227809454828,14.0999999999992,4.83063096365161));
#29327=CARTESIAN_POINT('Ctrl Pts',(-4.92436112622534,14.0592572834091,4.38730442774225));
#29328=CARTESIAN_POINT('Ctrl Pts',(-5.30932343282164,14.0202500034686,3.85744926888026));
#29329=CARTESIAN_POINT('Ctrl Pts',(-6.56268467750008,13.8932500034686,2.13234551188562));
#29330=CARTESIAN_POINT('Ctrl Pts',(-6.56268467749999,13.7662500034686,-5.55111512312578E-14));
#29331=CARTESIAN_POINT('Ctrl Pts',(-6.56268467749991,13.6392500034686,-2.13234551188562));
#29332=CARTESIAN_POINT('Ctrl Pts',(-5.30932343282153,13.5122500034687,-3.85744926888038));
#29333=CARTESIAN_POINT('Ctrl Pts',(-4.05596218814324,13.3852500034686,-5.58255302587488));
#29334=CARTESIAN_POINT('Ctrl Pts',(-2.0279810940716,13.2582500034686,-6.24148402692676));
#29335=CARTESIAN_POINT('Ctrl Pts',(0.,13.1312500034686,-6.90041502797853));
#29336=CARTESIAN_POINT('Ctrl Pts',(2.02798109407148,13.0042500034686,-6.24148402692676));
#29337=CARTESIAN_POINT('Ctrl Pts',(4.05596218814312,12.8772500034686,-5.58255302587488));
#29338=CARTESIAN_POINT('Ctrl Pts',(5.30932343282159,12.7502500034686,-3.85744926888038));
#29339=CARTESIAN_POINT('Ctrl Pts',(6.56268467750003,12.6232500034687,-2.13234551188562));
#29340=CARTESIAN_POINT('Ctrl Pts',(6.56268467749999,12.4962500034686,-5.55111512312578E-14));
#29341=CARTESIAN_POINT('',(4.81439089816027,14.0999999999991,4.45987336770942));
#29342=CARTESIAN_POINT('Origin',(-3.441691376338E-14,14.1,-1.15767576442529E-13));
#29343=CARTESIAN_POINT('Ctrl Pts',(4.81439089816027,14.0999999999991,4.45987336770942));
#29344=CARTESIAN_POINT('Ctrl Pts',(3.65313308585526,13.9950232909809,5.71344013542402));
#29345=CARTESIAN_POINT('Ctrl Pts',(2.0279810940716,13.8932500034686,6.24148402692665));
#29346=CARTESIAN_POINT('Ctrl Pts',(0.,13.7662500034686,6.90041502797853));
#29347=CARTESIAN_POINT('Ctrl Pts',(-2.02798109407165,13.6392500034685,6.24148402692665));
#29348=CARTESIAN_POINT('Ctrl Pts',(-4.05596218814318,13.5122500034686,5.58255302587488));
#29349=CARTESIAN_POINT('Ctrl Pts',(-5.30932343282153,13.3852500034687,3.85744926888026));
#29350=CARTESIAN_POINT('Ctrl Pts',(-6.56268467750003,13.2582500034686,2.13234551188562));
#29351=CARTESIAN_POINT('Ctrl Pts',(-6.56268467749999,13.1312500034686,-5.55111512312578E-14));
#29352=CARTESIAN_POINT('Ctrl Pts',(-6.56268467749997,13.0042500034686,-2.13234551188562));
#29353=CARTESIAN_POINT('Ctrl Pts',(-5.30932343282153,12.8772500034686,-3.85744926888038));
#29354=CARTESIAN_POINT('Ctrl Pts',(-4.05596218814312,12.7502500034686,-5.58255302587488));
#29355=CARTESIAN_POINT('Ctrl Pts',(-2.0279810940716,12.6232500034686,-6.24148402692676));
#29356=CARTESIAN_POINT('Ctrl Pts',(0.,12.4962500034686,-6.90041502797853));
#29357=CARTESIAN_POINT('Ctrl Pts',(2.0279810940716,12.3692500034686,-6.24148402692676));
#29358=CARTESIAN_POINT('Ctrl Pts',(4.05596218814318,12.2422500034686,-5.58255302587488));
#29359=CARTESIAN_POINT('Ctrl Pts',(5.30932343282159,12.1152500034687,-3.85744926888038));
#29360=CARTESIAN_POINT('Ctrl Pts',(6.56268467749997,11.9882500034686,-2.13234551188562));
#29361=CARTESIAN_POINT('Ctrl Pts',(6.56268467749999,11.8612500034686,-5.55111512312578E-14));
#29362=CARTESIAN_POINT('Origin',(0.,14.1,-5.55111512312578E-14));
#29363=CARTESIAN_POINT('',(-2.78947815484879E-8,0.272500004048667,7.93749999999994));
#29364=CARTESIAN_POINT('',(-3.45638790716338E-15,0.,7.93749999999994));
#29365=CARTESIAN_POINT('',(-3.55422631120848E-15,14.1,7.93749999999994));
#29366=CARTESIAN_POINT('',(-4.94987878329728,0.,6.20504683952217));
#29367=CARTESIAN_POINT('Origin',(0.,0.,0.));
#29368=CARTESIAN_POINT('Ctrl Pts',(-4.94987878329744,1.70436581514721E-14,
6.20504683952194));
#29369=CARTESIAN_POINT('Ctrl Pts',(-4.25667549292712,0.0458665906117807,
6.75802771916028));
#29370=CARTESIAN_POINT('Ctrl Pts',(-3.47565525918193,0.0917588069876965,
7.19098096194794));
#29371=CARTESIAN_POINT('Ctrl Pts',(-1.80587080516957,0.179620434800973,
7.77969428478989));
#29372=CARTESIAN_POINT('Ctrl Pts',(-0.929149370029642,0.224391358575233,
7.93232159581112));
#29373=CARTESIAN_POINT('Ctrl Pts',(-0.0302270880080657,0.270934936353027,
7.93745684009137));
#29374=CARTESIAN_POINT('Ctrl Pts',(-0.0151125175043377,0.271717524794004,
7.93749999994669));
#29375=CARTESIAN_POINT('Ctrl Pts',(-2.79692859872099E-8,0.272500005489119,
7.93749999999994));
#29376=CARTESIAN_POINT('Origin',(0.,14.1,-5.55111512312578E-14));
#29377=CARTESIAN_POINT('',(-7.49723371340113E-15,2.8125000069372,7.93749999999994));
#29378=CARTESIAN_POINT('',(-1.12431348720797E-14,2.49499999999995,7.93749999999994));
#29379=CARTESIAN_POINT('',(-3.55422631120848E-15,14.1,7.93749999999994));
#29380=CARTESIAN_POINT('',(0.88166725671843,0.000478964839786718,7.88808053401317));
#29381=CARTESIAN_POINT('Ctrl Pts',(-7.59808882477842E-15,2.49499999999995,
7.93749999999994));
#29382=CARTESIAN_POINT('Ctrl Pts',(-0.106534701701732,2.48948394341324,
7.93749999999994));
#29383=CARTESIAN_POINT('Ctrl Pts',(-0.21315395270652,2.48396350910906,7.93535520617803));
#29384=CARTESIAN_POINT('Ctrl Pts',(-1.34228594263562,2.42550034310937,7.88982662120746));
#29385=CARTESIAN_POINT('Ctrl Pts',(-2.34721168757627,2.37553557083703,7.65125568505704));
#29386=CARTESIAN_POINT('Ctrl Pts',(-4.22825870273555,2.27077151458366,6.79793705051727));
#29387=CARTESIAN_POINT('Ctrl Pts',(-5.08334996593937,2.21628774610785,6.18463094346842));
#29388=CARTESIAN_POINT('Ctrl Pts',(-6.5006440608075,2.11082869779532,4.67017498961196));
#29389=CARTESIAN_POINT('Ctrl Pts',(-7.05211470405572,2.06061785769598,3.78636421494984));
#29390=CARTESIAN_POINT('Ctrl Pts',(-7.78416468054134,1.95412820878321,1.86168514739494));
#29391=CARTESIAN_POINT('Ctrl Pts',(-7.95948874980504,1.90170675886746,0.839814635989911));
#29392=CARTESIAN_POINT('Ctrl Pts',(-7.91053560277102,1.79860647469392,-1.23798658579692));
#29393=CARTESIAN_POINT('Ctrl Pts',(-7.67720704198139,1.74387420518865,-2.27364806456493));
#29394=CARTESIAN_POINT('Ctrl Pts',(-6.8314704247939,1.63698339273262,-4.16953472439706));
#29395=CARTESIAN_POINT('Ctrl Pts',(-6.23671225204487,1.58759934630578,-5.01571954257537));
#29396=CARTESIAN_POINT('Ctrl Pts',(-4.75056903822628,1.48191850347762,-6.44270058120344));
#29397=CARTESIAN_POINT('Ctrl Pts',(-3.87038529466627,1.42787839297738,-7.00689205189505));
#29398=CARTESIAN_POINT('Ctrl Pts',(-1.93767034745183,1.32377210975524,-7.76748264468355));
#29399=CARTESIAN_POINT('Ctrl Pts',(-0.902962870018193,1.27175278765581,
-7.95444092917996));
#29400=CARTESIAN_POINT('Ctrl Pts',(1.16182405218545,1.16484413422693,-7.91845833154129));
#29401=CARTESIAN_POINT('Ctrl Pts',(2.17228416507604,1.11443142888325,-7.7027904396885));
#29402=CARTESIAN_POINT('Ctrl Pts',(4.07470078447887,1.01004914709921,-6.89142896184576));
#29403=CARTESIAN_POINT('Ctrl Pts',(4.94522720243699,0.95546296623569,-6.29600243658385));
#29404=CARTESIAN_POINT('Ctrl Pts',(6.39520826785213,0.84959255811601,-4.81301969746863));
#29405=CARTESIAN_POINT('Ctrl Pts',(6.96489277772095,0.79976927479356,-3.94386632210488));
#29406=CARTESIAN_POINT('Ctrl Pts',(7.74048137895843,0.693447126005146,-2.03673531687382));
#29407=CARTESIAN_POINT('Ctrl Pts',(7.93904769780024,0.640105599508897,-1.01701563326462));
#29408=CARTESIAN_POINT('Ctrl Pts',(7.9358969039521,0.537499009768316,1.06564198487979));
#29409=CARTESIAN_POINT('Ctrl Pts',(7.72452902037416,0.482767432371596,2.10842486523428));
#29410=CARTESIAN_POINT('Ctrl Pts',(6.91858062214297,0.375587045120146,4.02312003574284));
#29411=CARTESIAN_POINT('Ctrl Pts',(6.34250275689357,0.326128354483776,4.88107987113842));
#29412=CARTESIAN_POINT('Ctrl Pts',(4.98338043591633,0.227734503988947,6.24345275873069));
#29413=CARTESIAN_POINT('Ctrl Pts',(4.24352647010551,0.180775850154573,6.76810771789779));
#29414=CARTESIAN_POINT('Ctrl Pts',(2.62859963071464,0.0895653404014116,
7.54236428387094));
#29415=CARTESIAN_POINT('Ctrl Pts',(1.7666268132614,0.0464707913374984,7.78946812604573));
#29416=CARTESIAN_POINT('Ctrl Pts',(0.881700526094189,0.000651885411669714,
7.88837818770654));
#29417=CARTESIAN_POINT('Origin',(0.,0.,0.));
#29418=CARTESIAN_POINT('Ctrl Pts',(-2.79692896620887E-8,0.27250000548912,
7.93749999999994));
#29419=CARTESIAN_POINT('Ctrl Pts',(1.02412154774647,0.325526038068978,7.93750000360863));
#29420=CARTESIAN_POINT('Ctrl Pts',(2.0387743641584,0.376365153729017,7.73929238383186));
#29421=CARTESIAN_POINT('Ctrl Pts',(3.94831443777299,0.479964935848212,6.96344702576656));
#29422=CARTESIAN_POINT('Ctrl Pts',(4.82309953976759,0.53409799306983,6.38877090097829));
#29423=CARTESIAN_POINT('Ctrl Pts',(6.29329637177878,0.639639085112315,4.94443350923145));
#29424=CARTESIAN_POINT('Ctrl Pts',(6.87813000252512,0.689048938516753,4.09198074679249));
#29425=CARTESIAN_POINT('Ctrl Pts',(7.70277391587344,0.796096903334889,2.18604928342826));
#29426=CARTESIAN_POINT('Ctrl Pts',(7.9244674559821,0.850831949473949,1.14655097083738));
#29427=CARTESIAN_POINT('Ctrl Pts',(7.94912711678267,0.953674005975883,-0.933899729577854));
#29428=CARTESIAN_POINT('Ctrl Pts',(7.7614822973542,1.00656859984863,-1.95464195119927));
#29429=CARTESIAN_POINT('Ctrl Pts',(7.00634204924686,1.11297098466345,-3.87004642070044));
#29430=CARTESIAN_POINT('Ctrl Pts',(6.44520621813288,1.16296152304484,-4.74609739041746));
#29431=CARTESIAN_POINT('Ctrl Pts',(5.01056431745717,1.26864189885056,-6.24394855982245));
#29432=CARTESIAN_POINT('Ctrl Pts',(4.14726051728749,1.32318316370206,-6.84784030656768));
#29433=CARTESIAN_POINT('Ctrl Pts',(2.25484001253973,1.42774930414059,-7.67900151932538));
#29434=CARTESIAN_POINT('Ctrl Pts',(1.24697763497367,1.47793513664674,-7.90546715673995));
#29435=CARTESIAN_POINT('Ctrl Pts',(-0.818918926270186,1.58490124395344,
-7.96377300246748));
#29436=CARTESIAN_POINT('Ctrl Pts',(-1.85737939696264,1.63730526353135,-7.78731526484784));
#29437=CARTESIAN_POINT('Ctrl Pts',(-3.79840205169223,1.7411723140143,-7.0460200063592));
#29438=CARTESIAN_POINT('Ctrl Pts',(-4.68343537172677,1.79512128670165,-6.49149802903144));
#29439=CARTESIAN_POINT('Ctrl Pts',(-6.18410980182422,1.90092303841132,-5.08054464622637));
#29440=CARTESIAN_POINT('Ctrl Pts',(-6.78796368087669,1.95031103309894,-4.24012878133037));
#29441=CARTESIAN_POINT('Ctrl Pts',(-7.65293786749182,2.05705128565345,-2.35355027905519));
#29442=CARTESIAN_POINT('Ctrl Pts',(-7.89686305876648,2.11177478655014,-1.32150992259857));
#29443=CARTESIAN_POINT('Ctrl Pts',(-7.96799812014921,2.21510366089174,0.753726048810979));
#29444=CARTESIAN_POINT('Ctrl Pts',(-7.80391197499283,2.26712255178615,1.77660274747744));
#29445=CARTESIAN_POINT('Ctrl Pts',(-7.09294351488881,2.37368876670015,3.70968647754854));
#29446=CARTESIAN_POINT('Ctrl Pts',(-6.55030875033442,2.424129501784,4.60055434305804));
#29447=CARTESIAN_POINT('Ctrl Pts',(-5.14887517025208,2.52938034840208,6.12999929094172));
#29448=CARTESIAN_POINT('Ctrl Pts',(-4.30133144570552,2.58380545143214,6.75176605311574));
#29449=CARTESIAN_POINT('Ctrl Pts',(-2.4307452917941,2.68874131300215,7.62512804046215));
#29450=CARTESIAN_POINT('Ctrl Pts',(-1.42850359914185,2.73853625089095,7.87467129731538));
#29451=CARTESIAN_POINT('Ctrl Pts',(-0.270984323521069,2.79846922786978,
7.93403405453182));
#29452=CARTESIAN_POINT('Ctrl Pts',(-0.135428510124796,2.80548791309951,
7.93749999999994));
#29453=CARTESIAN_POINT('Ctrl Pts',(-8.32667268468867E-16,2.8125000069372,
7.93749999999994));
#29454=CARTESIAN_POINT('Origin',(0.,14.1,-5.55111512312578E-14));
#29455=CARTESIAN_POINT('',(1.10208006147732E-14,5.35250000693726,7.93749999999994));
#29456=CARTESIAN_POINT('',(-7.22738880307149E-15,5.03499999999995,7.93749999999994));
#29457=CARTESIAN_POINT('',(-3.55422631120848E-15,14.1,7.93749999999994));
#29458=CARTESIAN_POINT('Ctrl Pts',(-1.17961196366423E-15,5.03499999999995,
7.93749999999994));
#29459=CARTESIAN_POINT('Ctrl Pts',(-0.226056844747033,5.02329543493787,
7.93749999999994));
#29460=CARTESIAN_POINT('Ctrl Pts',(-0.452379981654991,5.01157708204239,
7.92784321473083));
#29461=CARTESIAN_POINT('Ctrl Pts',(-1.69853655960008,4.947054723693,7.82095339854726));
#29462=CARTESIAN_POINT('Ctrl Pts',(-2.6921904106198,4.89760386074584,7.53687454437464));
#29463=CARTESIAN_POINT('Ctrl Pts',(-4.52891436082978,4.79217528936648,6.60071567731681));
#29464=CARTESIAN_POINT('Ctrl Pts',(-5.35207911040713,4.73797561325999,5.95280125645727));
#29465=CARTESIAN_POINT('Ctrl Pts',(-6.70276294413308,4.63342744729077,4.37659409265729));
#29466=CARTESIAN_POINT('Ctrl Pts',(-7.21710810124169,4.58207327562376,3.46338007109142));
#29467=CARTESIAN_POINT('Ctrl Pts',(-7.86076483457757,4.47528268385131,1.50386890641363));
#29468=CARTESIAN_POINT('Ctrl Pts',(-7.98903928992562,4.42435921525472,0.47792817090558));
#29469=CARTESIAN_POINT('Ctrl Pts',(-7.84710502319438,4.3203471014793,-1.58817861604214));
#29470=CARTESIAN_POINT('Ctrl Pts',(-7.56954932656371,4.26569170997764,-2.60790862866832));
#29471=CARTESIAN_POINT('Ctrl Pts',(-6.64331468840853,4.15947748373841,-4.46390013422808));
#29472=CARTESIAN_POINT('Ctrl Pts',(-6.01020368526993,4.10989804615902,-5.28559000969115));
#29473=CARTESIAN_POINT('Ctrl Pts',(-4.46335320716717,4.00375460524552,-6.64421480518418));
#29474=CARTESIAN_POINT('Ctrl Pts',(-3.56337460212155,3.95013741324378,-7.16726464812353));
#29475=CARTESIAN_POINT('Ctrl Pts',(-1.59627750648389,3.84708629618733,-7.84586141832399));
#29476=CARTESIAN_POINT('Ctrl Pts',(-0.545802697038318,3.79326007407786,
-7.98800042731743));
#29477=CARTESIAN_POINT('Ctrl Pts',(1.5232931001589,3.6861283196508,-7.85689892133021));
#29478=CARTESIAN_POINT('Ctrl Pts',(2.52255243854008,3.63648678265965,-7.59526468261862));
#29479=CARTESIAN_POINT('Ctrl Pts',(4.38144464657043,3.53137005857384,-6.69986454385875));
#29480=CARTESIAN_POINT('Ctrl Pts',(5.22055929268208,3.4770168359775,-6.06885801179202));
#29481=CARTESIAN_POINT('Ctrl Pts',(6.60436711088727,3.37200380269381,-4.52296740072229));
#29482=CARTESIAN_POINT('Ctrl Pts',(7.13718103546469,3.32127619533951,-3.62429831056195));
#29483=CARTESIAN_POINT('Ctrl Pts',(7.82474966412857,3.21462848967094,-1.68195664241757));
#29484=CARTESIAN_POINT('Ctrl Pts',(7.97637434681364,3.16302331891095,-0.657989380878041));
#29485=CARTESIAN_POINT('Ctrl Pts',(7.88061997857165,3.05944882039942,1.414235300993));
#29486=CARTESIAN_POINT('Ctrl Pts',(7.62496599758344,3.00474205296789,2.44212492813196));
#29487=CARTESIAN_POINT('Ctrl Pts',(6.73866486039704,2.89817682906327,4.31821949312042));
#29488=CARTESIAN_POINT('Ctrl Pts',(6.12467717832555,2.84875338277315,5.15217888300741));
#29489=CARTESIAN_POINT('Ctrl Pts',(4.6079091059117,2.74282506352654,6.54514004824095));
#29490=CARTESIAN_POINT('Ctrl Pts',(3.71758504343212,2.68898434174957,7.08882301385243));
#29491=CARTESIAN_POINT('Ctrl Pts',(1.8675327906195,2.59070996736366,7.77156304982307));
#29492=CARTESIAN_POINT('Ctrl Pts',(0.937011186526622,2.54351571032439,7.93749999999995));
#29493=CARTESIAN_POINT('Ctrl Pts',(-9.57567358739198E-15,2.49499999999995,
7.93749999999994));
#29494=CARTESIAN_POINT('Ctrl Pts',(-4.16333634234434E-15,2.8125000069372,
7.93749999999994));
#29495=CARTESIAN_POINT('Ctrl Pts',(0.909721181897195,2.85960272030027,7.93749999999994));
#29496=CARTESIAN_POINT('Ctrl Pts',(1.81373654210814,2.90566668873107,7.78108663797075));
#29497=CARTESIAN_POINT('Ctrl Pts',(3.64424968482471,3.00226123805989,7.12664934258461));
#29498=CARTESIAN_POINT('Ctrl Pts',(4.5392362914694,3.05599840263424,6.59278652117131));
#29499=CARTESIAN_POINT('Ctrl Pts',(6.07041103374227,3.16203330133122,5.21615242755506));
#29500=CARTESIAN_POINT('Ctrl Pts',(6.69352650150149,3.21151668265289,4.38803538641356));
#29501=CARTESIAN_POINT('Ctrl Pts',(7.59893998270663,3.31791773142783,2.52148478176614));
#29502=CARTESIAN_POINT('Ctrl Pts',(7.86508648870957,3.37260318787555,1.4974371550653));
#29503=CARTESIAN_POINT('Ctrl Pts',(7.98292929617928,3.47639078088845,-0.571937970385089));
#29504=CARTESIAN_POINT('Ctrl Pts',(7.84247668327009,3.52765449298243,-1.59686075637627));
#29505=CARTESIAN_POINT('Ctrl Pts',(7.1759073479399,3.63437217351313,-3.54744652171663));
#29506=CARTESIAN_POINT('Ctrl Pts',(6.65191898932525,3.68538520334025,-4.45308697984317));
#29507=CARTESIAN_POINT('Ctrl Pts',(5.28394478157752,3.79017891575786,-6.01356419840023));
#29508=CARTESIAN_POINT('Ctrl Pts',(4.4524372569872,3.8444617038164,-6.65272668325208));
#29509=CARTESIAN_POINT('Ctrl Pts',(2.60411079213653,3.94973201136799,-7.56771579529136));
#29510=CARTESIAN_POINT('Ctrl Pts',(1.60753063476577,3.99926675237762,-7.84012292478179));
#29511=CARTESIAN_POINT('Ctrl Pts',(-0.46241352356521,4.1064424324734,-7.99354811436436));
#29512=CARTESIAN_POINT('Ctrl Pts',(-1.51649999363077,4.16075470053806,-7.8619566350794));
#29513=CARTESIAN_POINT('Ctrl Pts',(-3.49128361909894,4.2635449447295,-7.20251127690883));
#29514=CARTESIAN_POINT('Ctrl Pts',(-4.39558173765205,4.31705018290556,-6.68908533484584));
#29515=CARTESIAN_POINT('Ctrl Pts',(-5.95622232017642,4.42328254049896,-5.34651934819789));
#29516=CARTESIAN_POINT('Ctrl Pts',(-6.59818375596881,4.47297351342637,-4.53054689736886));
#29517=CARTESIAN_POINT('Ctrl Pts',(-7.54275895047591,4.57901622780737,-2.68399757361333));
#29518=CARTESIAN_POINT('Ctrl Pts',(-7.83034452991218,4.63363917585889,-1.66818531220936));
#29519=CARTESIAN_POINT('Ctrl Pts',(-7.99352465257869,4.73784241199925,0.394899491477628));
#29520=CARTESIAN_POINT('Ctrl Pts',(-7.87598550089385,4.78849377474384,1.4217173195101));
#29521=CARTESIAN_POINT('Ctrl Pts',(-7.25254590669157,4.89534568767877,3.38904270923797));
#29522=CARTESIAN_POINT('Ctrl Pts',(-6.74672145740871,4.94702620518506,4.30890979566154));
#29523=CARTESIAN_POINT('Ctrl Pts',(-5.4113035717782,5.05135240747281,5.89883540859768));
#29524=CARTESIAN_POINT('Ctrl Pts',(-4.59553406191032,5.10547343952972,6.55434440221265));
#29525=CARTESIAN_POINT('Ctrl Pts',(-2.76910942515123,5.21103367106865,7.50900517322945));
#29526=CARTESIAN_POINT('Ctrl Pts',(-1.77804029525862,5.26043825874281,7.80331188071559));
#29527=CARTESIAN_POINT('Ctrl Pts',(-0.505889512850405,5.32630652129486,
7.92542383965282));
#29528=CARTESIAN_POINT('Ctrl Pts',(-0.252793739486815,5.33941108333301,
7.93749999999994));
#29529=CARTESIAN_POINT('Ctrl Pts',(1.4363510381088E-14,5.35250000693726,
7.93749999999994));
#29530=CARTESIAN_POINT('Origin',(0.,14.1,-5.55111512312578E-14));
#29531=CARTESIAN_POINT('',(5.63434544398714E-15,7.89250000693726,7.93749999999994));
#29532=CARTESIAN_POINT('',(-2.2675240134523E-14,7.575,7.93749999999994));
#29533=CARTESIAN_POINT('',(-3.55422631120848E-15,14.1,7.93749999999994));
#29534=CARTESIAN_POINT('Ctrl Pts',(-4.73232564246473E-14,7.575,7.93749999999994));
#29535=CARTESIAN_POINT('Ctrl Pts',(-0.342311658315279,7.55727609926722,
7.93749999999994));
#29536=CARTESIAN_POINT('Ctrl Pts',(-0.68497495337198,7.53953399180717,7.91535684559342));
#29537=CARTESIAN_POINT('Ctrl Pts',(-2.04235410124708,7.46925285270692,7.73844696661338));
#29538=CARTESIAN_POINT('Ctrl Pts',(-3.0236112280855,7.41986896512291,7.41029951565781));
#29539=CARTESIAN_POINT('Ctrl Pts',(-4.82911112006103,7.31308036048196,6.38647618191546));
#29540=CARTESIAN_POINT('Ctrl Pts',(-5.63104004698734,7.25835344102439,5.69200889411091));
#29541=CARTESIAN_POINT('Ctrl Pts',(-6.90319245255078,7.1550961223596,4.05012740421005));
#29542=CARTESIAN_POINT('Ctrl Pts',(-7.36861551431731,7.10295295524148,3.12432227057014));
#29543=CARTESIAN_POINT('Ctrl Pts',(-7.92014358700705,6.99690506521083,1.14995909098138));
#29544=CARTESIAN_POINT('Ctrl Pts',(-8.00228782993313,6.94696459962651,0.120382632686124));
#29545=CARTESIAN_POINT('Ctrl Pts',(-7.76903905802668,6.84217723499278,-1.93179766506519));
#29546=CARTESIAN_POINT('Ctrl Pts',(-7.44860310515051,6.78770092206101,-2.9339584031999));
#29547=CARTESIAN_POINT('Ctrl Pts',(-6.44368460688526,6.6822691959813,-4.7484933656999));
#29548=CARTESIAN_POINT('Ctrl Pts',(-5.77228890485022,6.63202939067194,-5.54526016488532));
#29549=CARTESIAN_POINT('Ctrl Pts',(-4.16609576873437,6.52552939998956,-6.83392238043234));
#29550=CARTESIAN_POINT('Ctrl Pts',(-3.24782743689049,6.47316304583865,-7.31506224175719));
#29551=CARTESIAN_POINT('Ctrl Pts',(-1.25599959302191,6.37003200100285,-7.90767582300695));
#29552=CARTESIAN_POINT('Ctrl Pts',(-0.19894036866822,6.31530055290282,-8.00431738971416));
#29553=CARTESIAN_POINT('Ctrl Pts',(1.86512324238141,6.20842935041888,-7.78302404428111));
#29554=CARTESIAN_POINT('Ctrl Pts',(2.85332960957851,6.159046298985,-7.4774775956599));
#29555=CARTESIAN_POINT('Ctrl Pts',(4.66829436124367,6.05334902427052,-6.50254065466808));
#29556=CARTESIAN_POINT('Ctrl Pts',(5.47584795883197,5.99932067348471,-5.83876876716336));
#29557=CARTESIAN_POINT('Ctrl Pts',(6.79436786783019,5.89524572787936,-4.23384092563753));
#29558=CARTESIAN_POINT('Ctrl Pts',(7.29075169436021,5.84317694306221,-3.30664622040414));
#29559=CARTESIAN_POINT('Ctrl Pts',(7.8918229539737,5.73626051584764,-1.3307427956892));
#29560=CARTESIAN_POINT('Ctrl Pts',(7.997495578234,5.68587942536229,-0.302977384029888));
#29561=CARTESIAN_POINT('Ctrl Pts',(7.81082502569249,5.58147242770808,1.75661279939221));
#29562=CARTESIAN_POINT('Ctrl Pts',(7.51218622936447,5.52689184496292,2.76797332026668));
#29563=CARTESIAN_POINT('Ctrl Pts',(6.54735628589632,5.42104617759928,4.60393994857867));
#29564=CARTESIAN_POINT('Ctrl Pts',(5.89556966678131,5.371202341453,5.4135349757803));
#29565=CARTESIAN_POINT('Ctrl Pts',(4.31957594644649,5.26486945074441,6.73827251777554));
#29566=CARTESIAN_POINT('Ctrl Pts',(3.41055044889376,5.21158836949208,7.24090250175384));
#29567=CARTESIAN_POINT('Ctrl Pts',(1.64417149218024,5.1201304114449,7.8092239790489));
#29568=CARTESIAN_POINT('Ctrl Pts',(0.82385420015477,5.07765677112392,7.93749999999994));
#29569=CARTESIAN_POINT('Ctrl Pts',(-3.88578058618805E-15,5.03499999999995,
7.93749999999994));
#29570=CARTESIAN_POINT('Ctrl Pts',(1.12410081243297E-14,5.35250000693726,
7.93749999999994));
#29571=CARTESIAN_POINT('Ctrl Pts',(0.795747400676944,5.3937014898414,7.93749999999994));
#29572=CARTESIAN_POINT('Ctrl Pts',(1.58850203036173,5.43474801578022,7.8178277824124));
#29573=CARTESIAN_POINT('Ctrl Pts',(3.33309261958838,5.52507783561452,7.27674357940616));
#29574=CARTESIAN_POINT('Ctrl Pts',(4.24654561294269,5.57790716527978,6.7843777588313));
#29575=CARTESIAN_POINT('Ctrl Pts',(5.83699167769691,5.68432143404232,5.4768582264769));
#29576=CARTESIAN_POINT('Ctrl Pts',(6.49815399687296,5.73433953092022,4.67337969425469));
#29577=CARTESIAN_POINT('Ctrl Pts',(7.48220755546587,5.83999069856461,2.84760899648575));
#29578=CARTESIAN_POINT('Ctrl Pts',(7.79131248485743,5.89452468268523,1.84059542906963));
#29579=CARTESIAN_POINT('Ctrl Pts',(8.00030432227862,5.99911790400755,-0.215523862855896));
#29580=CARTESIAN_POINT('Ctrl Pts',(7.90590655801199,6.04927200587555,-1.24416836408562));
#29581=CARTESIAN_POINT('Ctrl Pts',(7.32610846746331,6.15624649883415,-3.22816302942619));
#29582=CARTESIAN_POINT('Ctrl Pts',(6.83871616481359,6.20871057345204,-4.16229300277298));
#29583=CARTESIAN_POINT('Ctrl Pts',(5.53627169395872,6.31254114570855,-5.78131711969542));
#29584=CARTESIAN_POINT('Ctrl Pts',(4.73656160992805,6.36647595409758,-6.45281104318585));
#29585=CARTESIAN_POINT('Ctrl Pts',(2.93255608983748,6.4722952489432,-7.44684143357893));
#29586=CARTESIAN_POINT('Ctrl Pts',(1.9470753922495,6.52168611371163,-7.76300370327744));
#29587=CARTESIAN_POINT('Ctrl Pts',(-0.114012506906427,6.62840324249997,
-8.00582976270103));
#29588=CARTESIAN_POINT('Ctrl Pts',(-1.1708829631323,6.6831249167361,-7.9205755090935));
#29589=CARTESIAN_POINT('Ctrl Pts',(-3.16718110901302,6.78648742079092,-7.35022657268397));
#29590=CARTESIAN_POINT('Ctrl Pts',(-4.08995031263565,6.83844847130781,-6.87963842497607));
#29591=CARTESIAN_POINT('Ctrl Pts',(-5.71088795218655,6.94502589301952,-5.60872603356154));
#29592=CARTESIAN_POINT('Ctrl Pts',(-6.39188199787461,6.99550338665362,-4.81828966055848));
#29593=CARTESIAN_POINT('Ctrl Pts',(-7.41688127095397,7.10078648989288,-3.01329749282044));
#29594=CARTESIAN_POINT('Ctrl Pts',(-7.74802851118764,7.15526953549469,-2.01448033935104));
#29595=CARTESIAN_POINT('Ctrl Pts',(-8.00418764143889,7.26072592251498,0.0438420911394408));
#29596=CARTESIAN_POINT('Ctrl Pts',(-7.93069937238232,7.31093956744832,1.08301320263485));
#29597=CARTESIAN_POINT('Ctrl Pts',(-7.3913569700335,7.4174302277125,3.07032729464053));
#29598=CARTESIAN_POINT('Ctrl Pts',(-6.93243106613093,7.46984628009873,4.00001582345517));
#29599=CARTESIAN_POINT('Ctrl Pts',(-5.6713126563452,7.57294957091596,5.65202322868132));
#29600=CARTESIAN_POINT('Ctrl Pts',(-4.8737152593873,7.62768176490096,6.35262566747103));
#29601=CARTESIAN_POINT('Ctrl Pts',(-3.07499434436709,7.73457066926074,7.38907513020429));
#29602=CARTESIAN_POINT('Ctrl Pts',(-2.0963984978319,7.78395459818715,7.72393351748084));
#29603=CARTESIAN_POINT('Ctrl Pts',(-0.722130494935735,7.85511019301398,
7.91288796105529));
#29604=CARTESIAN_POINT('Ctrl Pts',(-0.36089059047504,7.87381414320578,7.93749999999994));
#29605=CARTESIAN_POINT('Ctrl Pts',(2.15105711021124E-14,7.89250000693726,
7.93749999999994));
#29606=CARTESIAN_POINT('Origin',(0.,14.1,-5.55111512312578E-14));
#29607=CARTESIAN_POINT('',(1.93471957437057E-14,10.4325000069373,7.93749999999994));
#29608=CARTESIAN_POINT('',(-3.17393090743799E-14,10.115,7.93749999999994));
#29609=CARTESIAN_POINT('',(-3.55422631120848E-15,14.1,7.93749999999994));
#29610=CARTESIAN_POINT('Ctrl Pts',(-6.07847105982273E-14,10.115,7.93749999999995));
#29611=CARTESIAN_POINT('Ctrl Pts',(-0.458641069100447,10.0912529011698,
7.93749999999994));
#29612=CARTESIAN_POINT('Ctrl Pts',(-0.91749533059418,10.0674947638576,7.89774903451261));
#29613=CARTESIAN_POINT('Ctrl Pts',(-2.37949213000137,9.99179682744532,7.6413037997203));
#29614=CARTESIAN_POINT('Ctrl Pts',(-3.34393403904367,9.94221616601069,7.27114693454524));
#29615=CARTESIAN_POINT('Ctrl Pts',(-5.10235053238287,9.83506040630629,6.17045480967625));
#29616=CARTESIAN_POINT('Ctrl Pts',(-5.87355771397867,9.78097595121277,5.4414479144934));
#29617=CARTESIAN_POINT('Ctrl Pts',(-7.07550774143875,9.67806435335046,3.74210983253752));
#29618=CARTESIAN_POINT('Ctrl Pts',(-7.50109387229688,9.62450671837634,2.79277049347526));
#29619=CARTESIAN_POINT('Ctrl Pts',(-7.96502269082244,9.51831460222154,0.787015721554773));
#29620=CARTESIAN_POINT('Ctrl Pts',(-7.99990077643402,9.46867825178979,-0.250191428137116));
#29621=CARTESIAN_POINT('Ctrl Pts',(-7.66928610001285,9.36255558111798,-2.29785232778531));
#29622=CARTESIAN_POINT('Ctrl Pts',(-7.30005539978575,9.30791696570999,-3.28745464588663));
#29623=CARTESIAN_POINT('Ctrl Pts',(-6.21065675992449,9.2038011447894,-5.04781762740496));
#29624=CARTESIAN_POINT('Ctrl Pts',(-5.50824523766461,9.15302744259942,-5.80620494094393));
#29625=CARTESIAN_POINT('Ctrl Pts',(-3.84207252644146,9.04620348580589,-7.02295729521059));
#29626=CARTESIAN_POINT('Ctrl Pts',(-2.89078741216586,8.99467655318757,-7.46503428990422));
#29627=CARTESIAN_POINT('Ctrl Pts',(-0.873885938138244,8.89024726880558,
-7.95712065591083));
#29628=CARTESIAN_POINT('Ctrl Pts',(0.172096992937339,8.83608931891333,-8.0031079147963));
#29629=CARTESIAN_POINT('Ctrl Pts',(2.20968503930547,8.73058894406227,-7.69220686027878));
#29630=CARTESIAN_POINT('Ctrl Pts',(3.18266101044959,8.68116618949836,-7.34325526632608));
#29631=CARTESIAN_POINT('Ctrl Pts',(4.96692734416526,8.57407542163531,-6.28027790896194));
#29632=CARTESIAN_POINT('Ctrl Pts',(5.75524862147659,8.51934087651019,-5.56683073257915));
#29633=CARTESIAN_POINT('Ctrl Pts',(6.99294297133211,8.4165730217313,-3.89360469735698));
#29634=CARTESIAN_POINT('Ctrl Pts',(7.4381133042439,8.36353911669123,-2.95573212372524));
#29635=CARTESIAN_POINT('Ctrl Pts',(7.94623396652407,8.25716195000415,-0.960578242083116));
#29636=CARTESIAN_POINT('Ctrl Pts',(8.00370695894376,8.20722745802448,0.0778152885029483));
#29637=CARTESIAN_POINT('Ctrl Pts',(7.71675343248058,8.10148602972906,2.13192048341219));
#29638=CARTESIAN_POINT('Ctrl Pts',(7.36984710519358,8.04692986313322,3.12710210230098));
#29639=CARTESIAN_POINT('Ctrl Pts',(6.32112182604917,7.94242131969421,4.90865586491743));
#29640=CARTESIAN_POINT('Ctrl Pts',(5.63617464973127,7.89216652331995,5.68199097887513));
#29641=CARTESIAN_POINT('Ctrl Pts',(3.99521590435597,7.78521831887807,6.93752993327295));
#29642=CARTESIAN_POINT('Ctrl Pts',(3.05036582219345,7.73293905850887,7.40176912173894));
#29643=CARTESIAN_POINT('Ctrl Pts',(1.37502872996062,7.64619498305781,7.84798589621614));
#29644=CARTESIAN_POINT('Ctrl Pts',(0.68822505764354,7.61063428912565,7.93749999999995));
#29645=CARTESIAN_POINT('Ctrl Pts',(-5.06539254985228E-14,7.575,7.93749999999994));
#29646=CARTESIAN_POINT('Ctrl Pts',(2.2065682614425E-14,7.89250000693726,
7.93749999999994));
#29647=CARTESIAN_POINT('Ctrl Pts',(0.670234463880682,7.92720279551296,7.93749999999994));
#29648=CARTESIAN_POINT('Ctrl Pts',(1.33926411830421,7.96184320256437,7.8526050957819));
#29649=CARTESIAN_POINT('Ctrl Pts',(2.99899528290416,8.04777924853269,7.42256209273436));
#29650=CARTESIAN_POINT('Ctrl Pts',(3.94594229733037,8.09980337471834,6.96549066157424));
#29651=CARTESIAN_POINT('Ctrl Pts',(5.59508262861219,8.20671278851604,5.72248728462796));
#29652=CARTESIAN_POINT('Ctrl Pts',(6.28568674403704,8.25712238948963,4.95398167172491));
#29653=CARTESIAN_POINT('Ctrl Pts',(7.34761395585719,8.36150708669017,3.17923248220212));
#29654=CARTESIAN_POINT('Ctrl Pts',(7.70176239620213,8.41609272626145,2.185805446599));
#29655=CARTESIAN_POINT('Ctrl Pts',(8.0028739702793,8.52196072713378,0.133730110015611));
#29656=CARTESIAN_POINT('Ctrl Pts',(7.95274179886,8.57178599361545,-0.904289194325791));
#29657=CARTESIAN_POINT('Ctrl Pts',(7.45894724746318,8.6781091915952,-2.90300194306512));
#29658=CARTESIAN_POINT('Ctrl Pts',(7.02009311995133,8.73144480625242,-3.84461502766219));
#29659=CARTESIAN_POINT('Ctrl Pts',(5.79318113825769,8.83405446357269,-5.52748363661688));
#29660=CARTESIAN_POINT('Ctrl Pts',(5.0091654553918,8.88878612075992,-6.246762062927));
#29661=CARTESIAN_POINT('Ctrl Pts',(3.23158115468938,8.99596484558183,-7.32182655658592));
#29662=CARTESIAN_POINT('Ctrl Pts',(2.261178786054,9.04542275476233,-7.67719744432473));
#29663=CARTESIAN_POINT('Ctrl Pts',(0.225282078749181,9.15083555700256,-8.00187549109631));
#29664=CARTESIAN_POINT('Ctrl Pts',(-0.821676893795444,9.20504404347951,
-7.96276892182867));
#29665=CARTESIAN_POINT('Ctrl Pts',(-2.84136592469661,9.30961765943801,-7.48384049074501));
#29666=CARTESIAN_POINT('Ctrl Pts',(-3.79459828280301,9.36093547294504,-7.04856673754708));
#29667=CARTESIAN_POINT('Ctrl Pts',(-5.46846276992487,9.46771876164945,-5.84373748454541));
#29668=CARTESIAN_POINT('Ctrl Pts',(-6.17622004951641,9.51867553092367,-5.08994820655631));
#29669=CARTESIAN_POINT('Ctrl Pts',(-7.27801738319291,9.62266502984716,-3.33617908642261));
#29670=CARTESIAN_POINT('Ctrl Pts',(-7.65405982643817,9.67732382856,-2.34838016571328));
#29671=CARTESIAN_POINT('Ctrl Pts',(-7.99800884515637,9.783557562352,-0.302796444310101));
#29672=CARTESIAN_POINT('Ctrl Pts',(-7.9700067701409,9.83312568105443,0.734029790633371));
#29673=CARTESIAN_POINT('Ctrl Pts',(-7.51954531819447,9.93925837948954,2.7429537509967));
#29674=CARTESIAN_POINT('Ctrl Pts',(-7.09995207991095,9.99288819830642,3.69570617090967));
#29675=CARTESIAN_POINT('Ctrl Pts',(-5.90943326555059,10.0959691241069,5.4021971030452));
#29676=CARTESIAN_POINT('Ctrl Pts',(-5.14418327529678,10.1497406990643,6.13538192370205));
#29677=CARTESIAN_POINT('Ctrl Pts',(-3.39478789967035,10.2568671691636,7.24752814835039));
#29678=CARTESIAN_POINT('Ctrl Pts',(-2.43306750506007,10.3065228574942,7.62439934468818));
#29679=CARTESIAN_POINT('Ctrl Pts',(-0.954624042358646,10.3830723542333,
7.8944608539135));
#29680=CARTESIAN_POINT('Ctrl Pts',(-0.477232599070769,10.4077902928305,
7.93749999999994));
#29681=CARTESIAN_POINT('Ctrl Pts',(4.39925873507718E-14,10.4325000069373,
7.93749999999994));
#29682=CARTESIAN_POINT('Origin',(0.,14.1,-5.55111512312578E-14));
#29683=CARTESIAN_POINT('',(1.71352845339572E-14,12.9725000069373,7.93749999999994));
#29684=CARTESIAN_POINT('',(-2.6058228468434E-14,12.655,7.93749999999994));
#29685=CARTESIAN_POINT('',(-3.55422631120848E-15,14.1,7.93749999999994));
#29686=CARTESIAN_POINT('',(2.74837297199471,14.1000000000001,-7.44649932900082));
#29687=CARTESIAN_POINT('Ctrl Pts',(3.5527136788005E-14,12.9725000069373,
7.93749999999994));
#29688=CARTESIAN_POINT('Ctrl Pts',(0.441514761912383,12.9953603554592,7.93749999999994));
#29689=CARTESIAN_POINT('Ctrl Pts',(0.883293860395915,13.0182343905594,7.9006624651314));
#29690=CARTESIAN_POINT('Ctrl Pts',(2.33576268462579,13.093438996166,7.65557405604387));
#29691=CARTESIAN_POINT('Ctrl Pts',(3.30784468698389,13.1432450374237,7.28846560489659));
#29692=CARTESIAN_POINT('Ctrl Pts',(5.05761032906967,13.2495579450402,6.2035612026107));
#29693=CARTESIAN_POINT('Ctrl Pts',(5.81856026439151,13.3029516164402,5.49612540281248));
#29694=CARTESIAN_POINT('Ctrl Pts',(7.04227443491757,13.4055312000031,3.81060129369166));
#29695=CARTESIAN_POINT('Ctrl Pts',(7.48536577630057,13.4602620367625,2.84312496933517));
#29696=CARTESIAN_POINT('Ctrl Pts',(7.9610567611853,13.5674569903922,0.820826853952683));
#29697=CARTESIAN_POINT('Ctrl Pts',(8.00045927217651,13.6169227206054,-0.21180828650206));
#29698=CARTESIAN_POINT('Ctrl Pts',(7.68267872730624,13.7223187627277,-2.24888325280281));
#29699=CARTESIAN_POINT('Ctrl Pts',(7.32313231666238,13.7765364790642,-3.2330847874314));
#29700=CARTESIAN_POINT('Ctrl Pts',(6.32388253412427,13.8735480929797,-4.87847035940979));
#29701=CARTESIAN_POINT('Ctrl Pts',(5.7394996878338,13.9171161681885,-5.55419954457702));
#29702=CARTESIAN_POINT('Ctrl Pts',(4.36671516953879,14.0091367137029,-6.68835273608429));
#29703=CARTESIAN_POINT('Ctrl Pts',(3.58668621837271,14.0554678517837,-7.13709253708222));
#29704=CARTESIAN_POINT('Ctrl Pts',(2.74837297199447,14.1,-7.44649932900092));
#29705=CARTESIAN_POINT('',(-3.34416379519564,14.0999999999991,-7.19864395291942));
#29706=CARTESIAN_POINT('Origin',(0.,14.1,-5.55111512312578E-14));
#29707=CARTESIAN_POINT('Ctrl Pts',(-3.34416379519565,14.0999999999991,-7.19864395291943));
#29708=CARTESIAN_POINT('Ctrl Pts',(-2.53463385585193,14.0546446990372,-7.57471488127564));
#29709=CARTESIAN_POINT('Ctrl Pts',(-1.66747397020329,14.0113369458918,-7.81154239451509));
#29710=CARTESIAN_POINT('Ctrl Pts',(0.117776201608265,13.9189018912866,-7.98763914488592));
#29711=CARTESIAN_POINT('Ctrl Pts',(1.02330461842437,13.8720162670886,-7.92270143530879));
#29712=CARTESIAN_POINT('Ctrl Pts',(2.89294560306559,13.7752117019714,-7.46215127559449));
#29713=CARTESIAN_POINT('Ctrl Pts',(3.83066248839816,13.7243979284073,-7.02701411038719));
#29714=CARTESIAN_POINT('Ctrl Pts',(5.50073052807881,13.617582986142,-5.81591941690324));
#29715=CARTESIAN_POINT('Ctrl Pts',(6.21381880215461,13.566103830456,-5.04691532384178));
#29716=CARTESIAN_POINT('Ctrl Pts',(7.30246966856507,13.4616419945824,-3.27928268390965));
#29717=CARTESIAN_POINT('Ctrl Pts',(7.66803666025631,13.4074725272805,-2.29801717100145));
#29718=CARTESIAN_POINT('Ctrl Pts',(7.99895118058518,13.3019915132034,-0.263484125659655));
#29719=CARTESIAN_POINT('Ctrl Pts',(7.96619945483916,13.2525618377811,0.769599786611228));
#29720=CARTESIAN_POINT('Ctrl Pts',(7.50358141465413,13.1454511529384,2.79443427242162));
#29721=CARTESIAN_POINT('Ctrl Pts',(7.06711780140869,13.0907170380528,3.76413064667696));
#29722=CARTESIAN_POINT('Ctrl Pts',(5.85545454942371,12.9879843171251,5.45668017071748));
#29723=CARTESIAN_POINT('Ctrl Pts',(5.09981761461665,12.9348839510761,6.16879686335132));
#29724=CARTESIAN_POINT('Ctrl Pts',(3.35758310997936,12.828518746457,7.26578537214519));
#29725=CARTESIAN_POINT('Ctrl Pts',(2.38734373402949,12.7786097057428,7.63973996334981));
#29726=CARTESIAN_POINT('Ctrl Pts',(0.9184282191556,12.7025535383934,7.89766877418857));
#29727=CARTESIAN_POINT('Ctrl Pts',(0.459103976819018,12.6787710668436,7.93749999999995));
#29728=CARTESIAN_POINT('Ctrl Pts',(-4.413136522885E-14,12.655,7.93749999999994));
#29729=CARTESIAN_POINT('Origin',(100.349250287849,58.0000000000003,-5.55111512312578E-14));
#29730=CARTESIAN_POINT('',(93.7824240764952,63.3740766425393,-5.43873074039162E-14));
#29731=CARTESIAN_POINT('Origin',(97.7511740764953,56.5000000000003,-2.22044604925031E-13));
#29732=CARTESIAN_POINT('',(97.8805002878487,62.276000431186,-5.53448196339837E-14));
#29733=CARTESIAN_POINT('',(97.8805002878487,62.276000431186,-5.53448196339837E-14));
#29734=CARTESIAN_POINT('Origin',(100.349250287849,58.0000000000003,-5.55111512312578E-14));
#29735=CARTESIAN_POINT('Origin',(100.349250287849,58.0000000000003,-5.55111512312578E-14));
#29736=CARTESIAN_POINT('',(20.3135361207583,2.62592335746103,-5.57785450648505E-14));
#29737=CARTESIAN_POINT('',(12.3760361207582,16.3740766425391,-2.75518742664506E-14));
#29738=CARTESIAN_POINT('Origin',(16.3447861207583,9.50000000000001,-5.55111512312578E-14));
#29739=CARTESIAN_POINT('',(96.3805002878487,64.8740766425393,-5.52437573976652E-14));
#29740=CARTESIAN_POINT('Origin',(16.3447861207583,9.50000000000001,-5.55111512312578E-14));
#29741=CARTESIAN_POINT('Origin',(16.3447861207583,9.50000000000001,-5.55111512312578E-14));
#29742=CARTESIAN_POINT('',(16.215459909405,3.72399956881435,-5.60303715489411E-14));
#29743=CARTESIAN_POINT('',(20.3135361207583,2.62592335746103,-5.77226718584969E-14));
#29744=CARTESIAN_POINT('',(11.8805103239219,11.2323524991207,-3.23235249912074));
#29745=CARTESIAN_POINT('Origin',(13.746709909405,8.00000000000001,-5.55111512312578E-14));
#29746=CARTESIAN_POINT('',(12.1565117088869,13.8820812394808,-2.75430407740201));
#29747=CARTESIAN_POINT('Origin',(22.2987107739078,27.7500000031024,14.8125000036728));
#29748=CARTESIAN_POINT('',(12.0472108781263,14.1,-2.20150259211144));
#29749=CARTESIAN_POINT('Ctrl Pts',(12.0472108781263,14.1,-2.20150259211144));
#29750=CARTESIAN_POINT('Ctrl Pts',(12.0678843459318,14.0579048765951,-2.32254225822882));
#29751=CARTESIAN_POINT('Ctrl Pts',(12.0902925408505,14.0127946250959,-2.44179950334643));
#29752=CARTESIAN_POINT('Ctrl Pts',(12.1144581231571,13.9648546446133,-2.55934320764531));
#29753=CARTESIAN_POINT('Ctrl Pts',(12.1279271382907,13.9381346461283,-2.62485778585675));
#29754=CARTESIAN_POINT('Ctrl Pts',(12.1419425458387,13.9105347964401,-2.689840308819));
#29755=CARTESIAN_POINT('Ctrl Pts',(12.1565117088869,13.8820812394808,-2.75430407740201));
#29756=CARTESIAN_POINT('',(12.0472108781263,14.1,2.20150259211133));
#29757=CARTESIAN_POINT('Ctrl Pts',(12.0472108781263,14.1,2.20150259211132));
#29758=CARTESIAN_POINT('Ctrl Pts',(11.4907049197408,14.1,-6.03961325396085E-14));
#29759=CARTESIAN_POINT('Ctrl Pts',(12.0472108781263,14.1,-2.20150259211144));
#29760=CARTESIAN_POINT('',(12.1565117088869,13.8820812394808,2.7543040774019));
#29761=CARTESIAN_POINT('Ctrl Pts',(12.1565117088869,13.8820812394808,2.75430407740189));
#29762=CARTESIAN_POINT('Ctrl Pts',(12.1303722840449,13.9331315030524,2.6386456948073));
#29763=CARTESIAN_POINT('Ctrl Pts',(12.1060139372507,13.9814362147453,2.52131694964062));
#29764=CARTESIAN_POINT('Ctrl Pts',(12.0833998021185,14.0268345811549,2.40224286930925));
#29765=CARTESIAN_POINT('Ctrl Pts',(12.0707955071148,14.0521379765564,2.33587531525446));
#29766=CARTESIAN_POINT('Ctrl Pts',(12.058733515868,14.0765377118997,2.26896569206937));
#29767=CARTESIAN_POINT('Ctrl Pts',(12.0472108781263,14.1,2.20150259211132));
#29768=CARTESIAN_POINT('',(11.8805103239219,11.2323524991206,3.23235249912063));
#29769=CARTESIAN_POINT('Origin',(22.2987107722691,27.7500000007079,-14.8125000008489));
#29770=CARTESIAN_POINT('Origin',(13.746709909405,8.00000000000001,-5.55111512312578E-14));
#29771=CARTESIAN_POINT('Origin',(0.,14.1,-5.55111512312578E-14));
#29772=CARTESIAN_POINT('Ctrl Pts',(-4.21884749357559E-14,12.655,7.93749999999994));
#29773=CARTESIAN_POINT('Ctrl Pts',(-0.579914463779006,12.6249737179852,
7.93749999999994));
#29774=CARTESIAN_POINT('Ctrl Pts',(-1.15947748667141,12.5949656325551,7.87394595242885));
#29775=CARTESIAN_POINT('Ctrl Pts',(-2.72715977964003,12.5137956090803,7.52423713178313));
#29776=CARTESIAN_POINT('Ctrl Pts',(-3.67367098786041,12.4635073382784,7.11025260877252));
#29777=CARTESIAN_POINT('Ctrl Pts',(-5.37274800180185,12.3565676764149,5.93498728218027));
#29778=CARTESIAN_POINT('Ctrl Pts',(-6.1048637270787,12.3043463428722,5.17889833835055));
#29779=CARTESIAN_POINT('Ctrl Pts',(-7.23104489860743,12.200366936351,3.43325695867335));
#29780=CARTESIAN_POINT('Ctrl Pts',(-7.61663949860332,12.1463747744004,2.46209943522596));
#29781=CARTESIAN_POINT('Ctrl Pts',(-7.99150195866789,12.0406285218383,0.436459615612567));
#29782=CARTESIAN_POINT('Ctrl Pts',(-7.98103373474329,11.9912456527564,-0.598073328589007));
#29783=CARTESIAN_POINT('Ctrl Pts',(-7.56210694538478,11.8844344478724,-2.631022278771));
#29784=CARTESIAN_POINT('Ctrl Pts',(-7.14783970878105,11.8297061215808,-3.60781314121778));
#29785=CARTESIAN_POINT('Ctrl Pts',(-5.97652710178254,11.726482837202,-5.32343549253778));
#29786=CARTESIAN_POINT('Ctrl Pts',(-5.23858791367607,11.6742799952521,-6.05106074693906));
#29787=CARTESIAN_POINT('Ctrl Pts',(-3.52151821037508,11.5677490644444,-7.18813109666743));
#29788=CARTESIAN_POINT('Ctrl Pts',(-2.55747823859466,11.5174187748963,-7.58483040627315));
#29789=CARTESIAN_POINT('Ctrl Pts',(-0.522823087619294,11.4120702568272,
-7.98846239017354));
#29790=CARTESIAN_POINT('Ctrl Pts',(0.528861206991541,11.3576171069355,-7.98806497012856));
#29791=CARTESIAN_POINT('Ctrl Pts',(2.55402159520791,11.2527602000297,-7.58472519765813));
#29792=CARTESIAN_POINT('Ctrl Pts',(3.50954372789697,11.2028899408122,-7.19264619454136));
#29793=CARTESIAN_POINT('Ctrl Pts',(5.23841195128476,11.0958349775386,-6.05459635385751));
#29794=CARTESIAN_POINT('Ctrl Pts',(5.99012552771292,11.0427358686602,-5.31198777312635));
#29795=CARTESIAN_POINT('Ctrl Pts',(7.15451578954983,10.9392789840801,-3.58937238386304));
#29796=CARTESIAN_POINT('Ctrl Pts',(7.56035537425116,10.8854930493347,-2.62898080975064));
#29797=CARTESIAN_POINT('Ctrl Pts',(7.98007455387778,10.7795067290338,-0.613040650786056));
#29798=CARTESIAN_POINT('Ctrl Pts',(7.99240818396955,10.7300544630459,0.422884363461977));
#29799=CARTESIAN_POINT('Ctrl Pts',(7.61799584168553,10.6235764595768,2.46353045285619));
#29800=CARTESIAN_POINT('Ctrl Pts',(7.22640541893979,10.5688803811143,3.44703458659788));
#29801=CARTESIAN_POINT('Ctrl Pts',(6.09632292291776,10.4651907190041,5.18552436997988));
#29802=CARTESIAN_POINT('Ctrl Pts',(5.3763292293516,10.4137722115572,5.92874831387835));
#29803=CARTESIAN_POINT('Ctrl Pts',(3.68490340385191,10.3070866007226,7.10619693979162));
#29804=CARTESIAN_POINT('Ctrl Pts',(2.72725201401479,10.2562091665451,7.52586485362794));
#29805=CARTESIAN_POINT('Ctrl Pts',(1.15124096674424,10.174607904429,7.87484713432316));
#29806=CARTESIAN_POINT('Ctrl Pts',(0.575788488207968,10.144812651016,7.93749999999995));
#29807=CARTESIAN_POINT('Ctrl Pts',(-5.89805981832114E-14,10.115,7.93749999999994));
#29808=CARTESIAN_POINT('Ctrl Pts',(4.19109191795997E-14,10.4325000069373,
7.93749999999994));
#29809=CARTESIAN_POINT('Ctrl Pts',(0.557865244072069,10.4613846445709,7.93749999999994));
#29810=CARTESIAN_POINT('Ctrl Pts',(1.11551343313426,10.4902580437288,7.87868728685001));
#29811=CARTESIAN_POINT('Ctrl Pts',(2.67531963501286,10.5710202661449,7.54435003386203));
#29812=CARTESIAN_POINT('Ctrl Pts',(3.63494802025156,10.6217167186141,7.13173862549671));
#29813=CARTESIAN_POINT('Ctrl Pts',(5.33427756886483,10.728356179917,5.96668493147247));
#29814=CARTESIAN_POINT('Ctrl Pts',(6.05979254151313,10.7800024563114,5.22824691405044));
#29815=CARTESIAN_POINT('Ctrl Pts',(7.20259290222187,10.8835519868175,3.49673513528815));
#29816=CARTESIAN_POINT('Ctrl Pts',(7.60117704663546,10.9382608241988,2.51524429796514));
#29817=CARTESIAN_POINT('Ctrl Pts',(7.98930645957573,11.0448445082587,0.47690904840793));
#29818=CARTESIAN_POINT('Ctrl Pts',(7.98401058758636,11.0942627712914,-0.558596535002379));
#29819=CARTESIAN_POINT('Ctrl Pts',(7.57812242651015,11.200178396938,-2.57759503396377));
#29820=CARTESIAN_POINT('Ctrl Pts',(7.17850319392244,11.2540306452404,-3.54135438429488));
#29821=CARTESIAN_POINT('Ctrl Pts',(6.02588361859436,11.3576519189003,-5.27113262956091));
#29822=CARTESIAN_POINT('Ctrl Pts',(5.28023208431709,11.4104673366064,-6.01793109736661));
#29823=CARTESIAN_POINT('Ctrl Pts',(3.56056968016203,11.51748809768,-7.16752783866324));
#29824=CARTESIAN_POINT('Ctrl Pts',(2.60782998310456,11.5674741653522,-7.56639635070738));
#29825=CARTESIAN_POINT('Ctrl Pts',(0.584851620909866,11.6722180933054,-7.98425541389701));
#29826=CARTESIAN_POINT('Ctrl Pts',(-0.467546038531965,11.7267081791504,
-7.99198166929259));
#29827=CARTESIAN_POINT('Ctrl Pts',(-2.50478732152707,11.8321905996039,-7.60227911747851));
#29828=CARTESIAN_POINT('Ctrl Pts',(-3.47076794513677,11.8823769610477,-7.21265170917385));
#29829=CARTESIAN_POINT('Ctrl Pts',(-5.19568603346168,11.9888576904439,-6.08803326244125));
#29830=CARTESIAN_POINT('Ctrl Pts',(-5.93913557856266,12.0413268321481,-5.36522316328139));
#29831=CARTESIAN_POINT('Ctrl Pts',(-7.12304558585048,12.1444006137631,-3.65672997997241));
#29832=CARTESIAN_POINT('Ctrl Pts',(-7.54424276539696,12.1991335046262,-2.6820980975328));
#29833=CARTESIAN_POINT('Ctrl Pts',(-7.97679644286936,12.3060410559272,-0.651620238664076));
#29834=CARTESIAN_POINT('Ctrl Pts',(-7.9942243506473,12.35542632628,0.382469248486573));
#29835=CARTESIAN_POINT('Ctrl Pts',(-7.63307741991666,12.4610929734538,2.41094892881012));
#29836=CARTESIAN_POINT('Ctrl Pts',(-7.25371323229952,12.5151430945812,3.3853078408361));
#29837=CARTESIAN_POINT('Ctrl Pts',(-6.13923470871145,12.6192761720211,5.13787231059147));
#29838=CARTESIAN_POINT('Ctrl Pts',(-5.41307541922715,12.6712534316758,5.89802198140335));
#29839=CARTESIAN_POINT('Ctrl Pts',(-3.72307034122177,12.7781553778015,7.08453448555328));
#29840=CARTESIAN_POINT('Ctrl Pts',(-2.77930711107058,12.8285955790694,7.50515238039963));
#29841=CARTESIAN_POINT('Ctrl Pts',(-1.19600390162266,12.9105744081057,7.86986438990999));
#29842=CARTESIAN_POINT('Ctrl Pts',(-0.598244608684184,12.9415246434033,
7.93749999999995));
#29843=CARTESIAN_POINT('Ctrl Pts',(3.41393580072236E-14,12.9725000069373,
7.93749999999995));
#29844=CARTESIAN_POINT('Origin',(0.,14.1,-5.55111512312578E-14));
#29845=CARTESIAN_POINT('',(11.7464236222522,14.1,3.46459747903199));
#29846=CARTESIAN_POINT('Ctrl Pts',(12.1565117088871,13.8820812394807,2.75430407740162));
#29847=CARTESIAN_POINT('Ctrl Pts',(11.9496594695616,14.0046515569431,3.11258266557271));
#29848=CARTESIAN_POINT('Ctrl Pts',(11.7464236222522,14.1,3.46459747903198));
#29849=CARTESIAN_POINT('Origin',(0.,14.1,-5.55111512312578E-14));
#29850=CARTESIAN_POINT('Origin',(6.87335495470248,14.1000000000001,11.905));
#29851=CARTESIAN_POINT('',(13.7467099094049,2.29866609175239,0.));
#29852=CARTESIAN_POINT('Origin',(13.746709909405,8.,-5.26849434980831E-14));
#29853=CARTESIAN_POINT('',(8.87364124185536,14.1000000000001,8.44040252096795));
#29854=CARTESIAN_POINT('',(6.87335495470248,14.1000000000001,11.905));
#29855=CARTESIAN_POINT('',(6.87335495470248,12.6000000000002,11.905));
#29856=CARTESIAN_POINT('Ctrl Pts',(8.87364124185535,14.1,8.44040252096793));
#29857=CARTESIAN_POINT('Ctrl Pts',(7.93121327103568,13.6578583163328,10.0727356489016));
#29858=CARTESIAN_POINT('Ctrl Pts',(6.87335495470398,12.6000000000015,11.9049999999974));
#29859=CARTESIAN_POINT('',(6.87335495470248,1.5,11.9050000000001));
#29860=CARTESIAN_POINT('',(6.87335495470248,14.1000000000001,11.905));
#29861=CARTESIAN_POINT('',(8.8736412418553,2.22044604925031E-13,8.440402520968));
#29862=CARTESIAN_POINT('Ctrl Pts',(6.87335495470391,1.49999999999859,11.9049999999975));
#29863=CARTESIAN_POINT('Ctrl Pts',(7.93121327103561,0.442141683667228,10.0727356489018));
#29864=CARTESIAN_POINT('Ctrl Pts',(8.87364124185528,4.75454292391698E-14,
8.44040252096804));
#29865=CARTESIAN_POINT('',(11.7464236222521,0.,3.46459747903194));
#29866=CARTESIAN_POINT('',(6.87335495470248,1.11022302462516E-13,11.9050000000001));
#29867=CARTESIAN_POINT('',(13.746709909405,1.5,0.));
#29868=CARTESIAN_POINT('Ctrl Pts',(11.7464236222522,5.27371715124124E-14,
3.46459747903198));
#29869=CARTESIAN_POINT('Ctrl Pts',(12.6888515930718,0.442141683667233,1.83226435109827));
#29870=CARTESIAN_POINT('Ctrl Pts',(13.7467099094035,1.49999999999859,2.51795233061984E-12));
#29871=CARTESIAN_POINT('',(13.746709909405,14.1,-5.55111512312578E-14));
#29872=CARTESIAN_POINT('Origin',(13.746709909405,14.1,-5.55111512312578E-14));
#29873=CARTESIAN_POINT('',(11.7464236222523,14.1,-3.46459747903211));
#29874=CARTESIAN_POINT('Ctrl Pts',(11.7464236222523,14.1,-3.46459747903211));
#29875=CARTESIAN_POINT('Ctrl Pts',(11.8840862288804,14.0354153542157,-3.22615885004961));
#29876=CARTESIAN_POINT('Ctrl Pts',(12.0207522301902,13.9625255337105,-2.98944639211365));
#29877=CARTESIAN_POINT('Ctrl Pts',(12.1565117088869,13.8820812394808,-2.75430407740201));
#29878=CARTESIAN_POINT('Origin',(13.7467099094049,8.00000000000003,-1.4432899320127E-14));
#29879=CARTESIAN_POINT('',(11.7464236222521,0.,-3.46459747903194));
#29880=CARTESIAN_POINT('Ctrl Pts',(13.7467099094035,1.49999999999861,-2.52781374769102E-12));
#29881=CARTESIAN_POINT('Ctrl Pts',(12.6888515930719,0.442141683667257,-1.83226435109827));
#29882=CARTESIAN_POINT('Ctrl Pts',(11.7464236222522,7.62364532597791E-14,
-3.46459747903197));
#29883=CARTESIAN_POINT('',(8.8736412418553,0.,-8.440402520968));
#29884=CARTESIAN_POINT('',(13.746709909405,0.,0.));
#29885=CARTESIAN_POINT('',(6.87335495470243,1.49999999999995,-11.9050000000001));
#29886=CARTESIAN_POINT('Ctrl Pts',(8.87364124185533,4.80918128090362E-14,
-8.44040252096798));
#29887=CARTESIAN_POINT('Ctrl Pts',(7.93121327103565,0.442141683667221,-10.0727356489017));
#29888=CARTESIAN_POINT('Ctrl Pts',(6.87335495470394,1.49999999999859,-11.9049999999975));
#29889=CARTESIAN_POINT('',(6.87335495470248,12.6000000000001,-11.905));
#29890=CARTESIAN_POINT('',(6.87335495470248,14.1,-11.905));
#29891=CARTESIAN_POINT('',(8.8736412418553,14.1,-8.44040252096806));
#29892=CARTESIAN_POINT('Ctrl Pts',(6.87335495470396,12.6000000000015,-11.9049999999975));
#29893=CARTESIAN_POINT('Ctrl Pts',(7.93121327103563,13.6578583163328,-10.0727356489017));
#29894=CARTESIAN_POINT('Ctrl Pts',(8.87364124185529,14.1,-8.44040252096805));
#29895=CARTESIAN_POINT('',(13.746709909405,14.1,-5.55111512312578E-14));
#29896=CARTESIAN_POINT('Origin',(0.,14.1,-5.55111512312578E-14));
#29897=CARTESIAN_POINT('Origin',(0.,14.1,-5.55111512312578E-14));
#29898=CARTESIAN_POINT('',(2.87278238039673,14.0999999999999,-11.905));
#29899=CARTESIAN_POINT('Origin',(0.,14.1,-5.55111512312578E-14));
#29900=CARTESIAN_POINT('',(-2.87278238039679,14.1,-11.905));
#29901=CARTESIAN_POINT('',(0.,14.1,-11.905));
#29902=CARTESIAN_POINT('',(-8.87364124185536,14.1,-8.44040252096806));
#29903=CARTESIAN_POINT('Origin',(0.,14.1,-5.55111512312578E-14));
#29904=CARTESIAN_POINT('',(-11.7464236222523,14.1,-3.46459747903199));
#29905=CARTESIAN_POINT('',(-6.87335495470248,14.1,-11.905));
#29906=CARTESIAN_POINT('',(-11.7464236222523,14.1,3.46459747903199));
#29907=CARTESIAN_POINT('Origin',(0.,14.1,-5.55111512312578E-14));
#29908=CARTESIAN_POINT('',(-8.87364124185536,14.1000000000001,8.44040252096795));
#29909=CARTESIAN_POINT('',(-13.746709909405,14.1000000000001,-5.55111512312578E-14));
#29910=CARTESIAN_POINT('',(-2.87278238039679,14.1000000000001,11.905));
#29911=CARTESIAN_POINT('Origin',(0.,14.1,-5.55111512312578E-14));
#29912=CARTESIAN_POINT('',(2.87278238039668,14.1,11.905));
#29913=CARTESIAN_POINT('',(-6.87335495470248,14.1000000000001,11.905));
#29914=CARTESIAN_POINT('Origin',(0.,14.1,-5.55111512312578E-14));
#29915=CARTESIAN_POINT('Ctrl Pts',(4.81439089815928,14.1,4.45987336770828));
#29916=CARTESIAN_POINT('Ctrl Pts',(5.45085062221501,14.1,3.9043535918768));
#29917=CARTESIAN_POINT('Ctrl Pts',(5.88513855662796,14.1,3.30458855527548));
#29918=CARTESIAN_POINT('Ctrl Pts',(6.54523519250348,14.1,2.178289565022));
#29919=CARTESIAN_POINT('Ctrl Pts',(6.81015684136435,14.1,1.49685119003521));
#29920=CARTESIAN_POINT('Ctrl Pts',(7.07650468880845,14.1,0.257408185061271));
#29921=CARTESIAN_POINT('Ctrl Pts',(7.11305348659363,14.1000000000836,-0.220388032780179));
#29922=CARTESIAN_POINT('Ctrl Pts',(7.12185249698299,14.1000000000836,-1.09051005975987));
#29923=CARTESIAN_POINT('Ctrl Pts',(7.08061887026275,14.0999999999992,-1.56201229863969));
#29924=CARTESIAN_POINT('Ctrl Pts',(6.9072264798878,14.0999999999992,-2.49066379795867));
#29925=CARTESIAN_POINT('Ctrl Pts',(6.77543880742199,14.1,-2.94553773574212));
#29926=CARTESIAN_POINT('Ctrl Pts',(6.51181911719829,14.1,-3.60682978802007));
#29927=CARTESIAN_POINT('Ctrl Pts',(6.41224112310757,14.1,-3.82471112630172));
#29928=CARTESIAN_POINT('Ctrl Pts',(6.10972373678835,14.1,-4.40864758554243));
#29929=CARTESIAN_POINT('Ctrl Pts',(5.8837428763729,14.1,-4.76492359630792));
#29930=CARTESIAN_POINT('Ctrl Pts',(5.26565977805594,14.1,-5.58908540006088));
#29931=CARTESIAN_POINT('Ctrl Pts',(4.83647382882801,14.1,-6.03739008948846));
#29932=CARTESIAN_POINT('Ctrl Pts',(3.86571978096819,14.1,-6.83377631056592));
#29933=CARTESIAN_POINT('Ctrl Pts',(3.32495245618938,14.1,-7.17528491172701));
#29934=CARTESIAN_POINT('Ctrl Pts',(2.74837297199472,14.1,-7.44649932900086));
#29935=CARTESIAN_POINT('Ctrl Pts',(-3.34416379519642,14.1,-7.19864395292077));
#29936=CARTESIAN_POINT('Ctrl Pts',(-3.80496175909537,14.1,-6.93317036127327));
#29937=CARTESIAN_POINT('Ctrl Pts',(-4.23728703671821,14.1,-6.62113500445306));
#29938=CARTESIAN_POINT('Ctrl Pts',(-5.02490897558888,14.1,-5.91942515123866));
#29939=CARTESIAN_POINT('Ctrl Pts',(-5.37929764729192,14.1,-5.53294123412414));
#29940=CARTESIAN_POINT('Ctrl Pts',(-5.90207512304697,14.1,-4.83255037860479));
#29941=CARTESIAN_POINT('Ctrl Pts',(-6.09621395038283,14.1,-4.53270849908774));
#29942=CARTESIAN_POINT('Ctrl Pts',(-6.73632890639296,14.1,-3.36860941126136));
#29943=CARTESIAN_POINT('Ctrl Pts',(-7.03116378822683,14.0999999999992,-2.42871440474076));
#29944=CARTESIAN_POINT('Ctrl Pts',(-7.21129158371066,14.0999999999992,-0.716849514103212));
#29945=CARTESIAN_POINT('Ctrl Pts',(-7.20260496870702,14.0999999999998,0.25667633591363));
#29946=CARTESIAN_POINT('Ctrl Pts',(-6.67217509398093,14.0999999999998,2.0265111548136));
#29947=CARTESIAN_POINT('Ctrl Pts',(-6.35366664533318,14.1,2.68669863016612));
#29948=CARTESIAN_POINT('Ctrl Pts',(-5.58382739346403,14.1,3.7930184173696));
#29949=CARTESIAN_POINT('Ctrl Pts',(-5.10184834759149,14.1,4.34342875622177));
#29950=CARTESIAN_POINT('Ctrl Pts',(-4.44227809454922,14.1,4.83063096365287));
#29951=CARTESIAN_POINT('Origin',(0.,0.,0.));
#29952=CARTESIAN_POINT('',(2.87278238039684,1.11022302462516E-13,11.9050000000001));
#29953=CARTESIAN_POINT('Origin',(0.,0.,0.));
#29954=CARTESIAN_POINT('',(-2.87278238039695,1.11022302462516E-13,11.9050000000001));
#29955=CARTESIAN_POINT('',(-6.87335495470248,1.11022302462516E-13,11.9050000000001));
#29956=CARTESIAN_POINT('',(-8.87364124185519,1.66533453693773E-13,8.440402520968));
#29957=CARTESIAN_POINT('Origin',(0.,0.,0.));
#29958=CARTESIAN_POINT('',(-11.7464236222522,0.,3.46459747903194));
#29959=CARTESIAN_POINT('',(-13.746709909405,0.,0.));
#29960=CARTESIAN_POINT('',(-11.7464236222522,0.,-3.46459747903194));
#29961=CARTESIAN_POINT('Origin',(0.,0.,0.));
#29962=CARTESIAN_POINT('',(-8.87364124185519,0.,-8.44040252096812));
#29963=CARTESIAN_POINT('',(-6.87335495470248,-1.11022302462516E-13,-11.9050000000001));
#29964=CARTESIAN_POINT('',(-2.87278238039701,0.,-11.9050000000001));
#29965=CARTESIAN_POINT('Origin',(0.,0.,0.));
#29966=CARTESIAN_POINT('',(2.87278238039684,0.,-11.9050000000001));
#29967=CARTESIAN_POINT('',(6.87335495470248,0.,-11.9050000000001));
#29968=CARTESIAN_POINT('Origin',(0.,0.,0.));
#29969=CARTESIAN_POINT('Origin',(0.,0.,0.));
#29970=CARTESIAN_POINT('Ctrl Pts',(5.75296004380522,2.01337031627161E-17,
-3.15789184594319));
#29971=CARTESIAN_POINT('Ctrl Pts',(6.16805145920931,1.85363260495959E-17,
-2.56166546672911));
#29972=CARTESIAN_POINT('Ctrl Pts',(6.48269012589373,1.53992749440315E-15,
-1.90162976751356));
#29973=CARTESIAN_POINT('Ctrl Pts',(6.93094848290557,1.53992749440315E-15,
-0.352314338723844));
#29974=CARTESIAN_POINT('Ctrl Pts',(6.9735621303957,-2.29033109896044E-15,
0.431250662897198));
#29975=CARTESIAN_POINT('Ctrl Pts',(6.89132306443144,-2.30578919340332E-15,
1.96534646388369));
#29976=CARTESIAN_POINT('Ctrl Pts',(6.67510037401339,1.07986803510167E-13,
2.84128554352015));
#29977=CARTESIAN_POINT('Ctrl Pts',(6.07641308406255,1.07959211142374E-13,
4.14593238259473));
#29978=CARTESIAN_POINT('Ctrl Pts',(5.82171281817818,-4.17642667584523E-16,
4.55202544384661));
#29979=CARTESIAN_POINT('Ctrl Pts',(5.01566141664707,-4.30629552179204E-16,
5.67172768687367));
#29980=CARTESIAN_POINT('Ctrl Pts',(4.29205372561275,3.00713586736219E-16,
6.34879214397254));
#29981=CARTESIAN_POINT('Ctrl Pts',(2.52623730895339,2.62449789740603E-16,
7.45004618249224));
#29982=CARTESIAN_POINT('Ctrl Pts',(1.61227135251105,-2.22244929069149E-16,
7.73897430176318));
#29983=CARTESIAN_POINT('Ctrl Pts',(0.881575105385269,-2.28428747016988E-16,
7.88725607656427));
#29984=CARTESIAN_POINT('Ctrl Pts',(-4.94987878329725,-1.12418580016597E-16,
6.20504683952215));
#29985=CARTESIAN_POINT('Ctrl Pts',(-5.27029315480931,-1.12342428493602E-16,
5.89885818333482));
#29986=CARTESIAN_POINT('Ctrl Pts',(-5.564488656497,-2.81302745768979E-16,
5.56638595682626));
#29987=CARTESIAN_POINT('Ctrl Pts',(-6.09390465339696,-2.81302745768979E-16,
4.85636985748995));
#29988=CARTESIAN_POINT('Ctrl Pts',(-6.33453362765511,5.20414605987702E-11,
4.47177250256802));
#29989=CARTESIAN_POINT('Ctrl Pts',(-6.66809651486317,5.20414672868805E-11,
3.81063946212714));
#29990=CARTESIAN_POINT('Ctrl Pts',(-6.78350940590364,-1.77077700830533E-16,
3.54465253981978));
#29991=CARTESIAN_POINT('Ctrl Pts',(-7.21722783075047,-1.77077700830533E-16,
2.36186655823779));
#29992=CARTESIAN_POINT('Ctrl Pts',(-7.37128688497629,9.00446286223025E-16,
1.39508370515086));
#29993=CARTESIAN_POINT('Ctrl Pts',(-7.32878830602581,9.11740271284661E-16,
0.197855159856712));
#29994=CARTESIAN_POINT('Ctrl Pts',(-7.31012622920285,1.01089725039356E-13,
-0.0350591557617014));
#29995=CARTESIAN_POINT('Ctrl Pts',(-7.16601113065448,1.0110022688177E-13,
-1.13639635415202));
#29996=CARTESIAN_POINT('Ctrl Pts',(-6.89059191747676,6.30023822827895E-16,
-1.97852215970624));
#29997=CARTESIAN_POINT('Ctrl Pts',(-6.28104839707265,6.4286537953397E-16,
-3.08791508612891));
#29998=CARTESIAN_POINT('Ctrl Pts',(-6.06694326657524,-1.73558303903062E-11,
-3.41136766122037));
#29999=CARTESIAN_POINT('Ctrl Pts',(-5.64873030316675,-1.73558168339861E-11,
-3.94251068996791));
#30000=CARTESIAN_POINT('Ctrl Pts',(-5.45210843203702,-8.46568959619048E-16,
-4.16357330811727));
#30001=CARTESIAN_POINT('Ctrl Pts',(-4.64607031268313,-8.23624923925226E-16,
-4.95292977127109));
#30002=CARTESIAN_POINT('Ctrl Pts',(-3.94675564135096,-2.57359874551289E-17,
-5.41802989602537));
#30003=CARTESIAN_POINT('Ctrl Pts',(-3.17934379362958,-1.79845011350651E-17,
-5.74113257277705));
#30004=CARTESIAN_POINT('Origin',(6.87335495470248,14.1,-11.905));
#30005=CARTESIAN_POINT('',(-6.87335495470248,12.6,-11.905));
#30006=CARTESIAN_POINT('',(-6.87335495470254,1.49999999999995,-11.9050000000001));
#30007=CARTESIAN_POINT('',(-6.87335495470248,14.1,-11.905));
#30008=CARTESIAN_POINT('Ctrl Pts',(-6.87335495469956,12.6000000000015,-11.905));
#30009=CARTESIAN_POINT('Ctrl Pts',(-4.75763832203614,13.6578583163329,-11.905));
#30010=CARTESIAN_POINT('Ctrl Pts',(-2.87278238039677,14.1000000000001,-11.905));
#30011=CARTESIAN_POINT('Ctrl Pts',(2.87278238039676,14.1000000000001,-11.905));
#30012=CARTESIAN_POINT('Ctrl Pts',(4.75763832203614,13.6578583163329,-11.905));
#30013=CARTESIAN_POINT('Ctrl Pts',(6.87335495469956,12.6000000000015,-11.905));
#30014=CARTESIAN_POINT('Ctrl Pts',(6.87335495469949,1.49999999999853,-11.905));
#30015=CARTESIAN_POINT('Ctrl Pts',(4.75763832203613,0.442141683667185,-11.905));
#30016=CARTESIAN_POINT('Ctrl Pts',(2.87278238039681,1.09299837331425E-14,
-11.905));
#30017=CARTESIAN_POINT('Ctrl Pts',(-2.87278238039699,2.69150849428633E-14,
-11.905));
#30018=CARTESIAN_POINT('Ctrl Pts',(-4.75763832203628,0.442141683667205,
-11.905));
#30019=CARTESIAN_POINT('Ctrl Pts',(-6.87335495469961,1.49999999999853,-11.905));
#30020=CARTESIAN_POINT('Origin',(-6.87335495470248,14.1,-11.905));
#30021=CARTESIAN_POINT('',(-13.746709909405,12.6000000000001,-5.55111512312578E-14));
#30022=CARTESIAN_POINT('',(-13.746709909405,1.5,0.));
#30023=CARTESIAN_POINT('',(-13.746709909405,14.1000000000001,-5.55111512312578E-14));
#30024=CARTESIAN_POINT('Ctrl Pts',(-13.7467099094035,12.6000000000015,-2.58585423657939E-12));
#30025=CARTESIAN_POINT('Ctrl Pts',(-12.6888515930718,13.6578583163328,-1.83226435109829));
#30026=CARTESIAN_POINT('Ctrl Pts',(-11.7464236222522,14.1,-3.46459747903196));
#30027=CARTESIAN_POINT('Ctrl Pts',(-8.87364124185531,14.1,-8.44040252096801));
#30028=CARTESIAN_POINT('Ctrl Pts',(-7.93121327103563,13.6578583163329,-10.0727356489017));
#30029=CARTESIAN_POINT('Ctrl Pts',(-6.87335495470392,12.6000000000015,-11.9049999999975));
#30030=CARTESIAN_POINT('Ctrl Pts',(-6.87335495470394,1.49999999999851,-11.9049999999975));
#30031=CARTESIAN_POINT('Ctrl Pts',(-7.93121327103559,0.442141683667188,
-10.0727356489018));
#30032=CARTESIAN_POINT('Ctrl Pts',(-8.87364124185522,2.73249593328561E-16,
-8.44040252096814));
#30033=CARTESIAN_POINT('Ctrl Pts',(-11.7464236222522,-3.702531989602E-14,
-3.46459747903195));
#30034=CARTESIAN_POINT('Ctrl Pts',(-12.6888515930719,0.442141683667145,
-1.83226435109824));
#30035=CARTESIAN_POINT('Ctrl Pts',(-13.7467099094036,1.49999999999851,-2.48312588068041E-12));
#30036=CARTESIAN_POINT('Origin',(-13.746709909405,14.1000000000001,-5.55111512312578E-14));
#30037=CARTESIAN_POINT('',(-6.87335495470248,12.6000000000001,11.905));
#30038=CARTESIAN_POINT('',(-6.87335495470254,1.50000000000011,11.9050000000001));
#30039=CARTESIAN_POINT('',(-6.87335495470248,14.1000000000001,11.905));
#30040=CARTESIAN_POINT('Ctrl Pts',(-6.87335495470397,12.6000000000014,11.9049999999975));
#30041=CARTESIAN_POINT('Ctrl Pts',(-7.93121327103568,13.6578583163328,10.0727356489017));
#30042=CARTESIAN_POINT('Ctrl Pts',(-8.87364124185536,14.1,8.44040252096793));
#30043=CARTESIAN_POINT('Ctrl Pts',(-11.7464236222522,14.1,3.46459747903198));
#30044=CARTESIAN_POINT('Ctrl Pts',(-12.6888515930718,13.6578583163328,1.83226435109828));
#30045=CARTESIAN_POINT('Ctrl Pts',(-13.7467099094035,12.6000000000015,2.54058002098945E-12));
#30046=CARTESIAN_POINT('Ctrl Pts',(-13.7467099094036,1.49999999999852,2.48196499901576E-12));
#30047=CARTESIAN_POINT('Ctrl Pts',(-12.6888515930719,0.442141683667162,
1.83226435109823));
#30048=CARTESIAN_POINT('Ctrl Pts',(-11.7464236222522,-2.11768434829634E-14,
3.46459747903193));
#30049=CARTESIAN_POINT('Ctrl Pts',(-8.87364124185527,-5.19174227324266E-15,
8.44040252096809));
#30050=CARTESIAN_POINT('Ctrl Pts',(-7.9312132710356,0.442141683667188,10.0727356489018));
#30051=CARTESIAN_POINT('Ctrl Pts',(-6.87335495470391,1.49999999999856,11.9049999999975));
#30052=CARTESIAN_POINT('Origin',(-6.87335495470248,14.1000000000001,11.905));
#30053=CARTESIAN_POINT('Ctrl Pts',(6.87335495469949,12.6000000000015,11.905));
#30054=CARTESIAN_POINT('Ctrl Pts',(4.75763832203604,13.6578583163328,11.905));
#30055=CARTESIAN_POINT('Ctrl Pts',(2.87278238039665,14.1,11.905));
#30056=CARTESIAN_POINT('Ctrl Pts',(-2.87278238039675,14.1,11.905));
#30057=CARTESIAN_POINT('Ctrl Pts',(-4.75763832203612,13.6578583163328,11.905));
#30058=CARTESIAN_POINT('Ctrl Pts',(-6.87335495469954,12.6000000000015,11.905));
#30059=CARTESIAN_POINT('Ctrl Pts',(-6.87335495469967,1.49999999999856,11.905));
#30060=CARTESIAN_POINT('Ctrl Pts',(-4.75763832203629,0.442141683667203,
11.905));
#30061=CARTESIAN_POINT('Ctrl Pts',(-2.87278238039696,1.99472203129849E-14,
11.905));
#30062=CARTESIAN_POINT('Ctrl Pts',(2.87278238039686,1.99472203129849E-14,
11.905));
#30063=CARTESIAN_POINT('Ctrl Pts',(4.75763832203619,0.442141683667202,11.905));
#30064=CARTESIAN_POINT('Ctrl Pts',(6.87335495469956,1.49999999999856,11.905));
#30065=CARTESIAN_POINT('Origin',(-5.55111512312578E-14,1.5,0.));
#30066=CARTESIAN_POINT('Origin',(-5.55111512312578E-14,1.5,0.));
#30067=CARTESIAN_POINT('Origin',(0.,14.1,-5.55111512312578E-14));
#30068=CARTESIAN_POINT('Origin',(0.,14.1,-5.55111512312578E-14));
#30069=CARTESIAN_POINT('Origin',(-5.55111512312578E-14,1.5,0.));
#30070=CARTESIAN_POINT('Origin',(0.,14.1,-5.55111512312578E-14));
#30071=CARTESIAN_POINT('Origin',(-5.55111512312578E-14,1.5,0.));
#30072=CARTESIAN_POINT('Origin',(0.,14.1,-5.55111512312578E-14));
#30073=CARTESIAN_POINT('Origin',(-5.55111512312578E-14,1.5,0.));
#30074=CARTESIAN_POINT('Origin',(0.,14.1,-5.55111512312578E-14));
#30075=CARTESIAN_POINT('Origin',(-5.55111512312578E-14,1.5,0.));
#30076=CARTESIAN_POINT('Origin',(0.,14.1,-5.55111512312578E-14));
#30077=CARTESIAN_POINT('Ctrl Pts',(-6.56268467749999,16.3062500034686,-5.55111512312578E-14));
#30078=CARTESIAN_POINT('Ctrl Pts',(-6.56268467750003,16.1792500034687,-2.13234551188562));
#30079=CARTESIAN_POINT('Ctrl Pts',(-5.30932343282159,16.0522500034687,-3.85744926888038));
#30080=CARTESIAN_POINT('Ctrl Pts',(-4.05596218814306,15.9252500034686,-5.58255302587488));
#30081=CARTESIAN_POINT('Ctrl Pts',(-2.0279810940716,15.7982500034687,-6.24148402692676));
#30082=CARTESIAN_POINT('Ctrl Pts',(-1.1673575708729E-13,15.6712500034687,
-6.90041502797853));
#30083=CARTESIAN_POINT('Ctrl Pts',(2.02798109407148,15.5442500034687,-6.24148402692676));
#30084=CARTESIAN_POINT('Ctrl Pts',(4.05596218814312,15.4172500034687,-5.58255302587488));
#30085=CARTESIAN_POINT('Ctrl Pts',(5.30932343282159,15.2902500034686,-3.85744926888038));
#30086=CARTESIAN_POINT('Ctrl Pts',(6.56268467750008,15.1632500034687,-2.13234551188562));
#30087=CARTESIAN_POINT('Ctrl Pts',(6.56268467749999,15.0362500034686,-5.55111512312578E-14));
#30088=CARTESIAN_POINT('Ctrl Pts',(6.56268467750003,14.9092500034686,2.13234551188562));
#30089=CARTESIAN_POINT('Ctrl Pts',(5.30932343282159,14.7822500034687,3.85744926888026));
#30090=CARTESIAN_POINT('Ctrl Pts',(4.05596218814318,14.6552500034686,5.58255302587488));
#30091=CARTESIAN_POINT('Ctrl Pts',(2.0279810940716,14.5282500034686,6.24148402692665));
#30092=CARTESIAN_POINT('Ctrl Pts',(0.,14.4012500034686,6.90041502797853));
#30093=CARTESIAN_POINT('Ctrl Pts',(-2.02798109407154,14.2742500034686,6.24148402692665));
#30094=CARTESIAN_POINT('Ctrl Pts',(-4.05596218814312,14.1472500034686,5.58255302587488));
#30095=CARTESIAN_POINT('Ctrl Pts',(-5.30932343282164,14.0202500034686,3.85744926888026));
#30096=CARTESIAN_POINT('Ctrl Pts',(-6.56268467750008,13.8932500034686,2.13234551188562));
#30097=CARTESIAN_POINT('Ctrl Pts',(-6.56268467749999,13.7662500034686,-5.55111512312578E-14));
#30098=CARTESIAN_POINT('Ctrl Pts',(-6.56268467749991,13.6392500034686,-2.13234551188562));
#30099=CARTESIAN_POINT('Ctrl Pts',(-5.30932343282153,13.5122500034687,-3.85744926888038));
#30100=CARTESIAN_POINT('Ctrl Pts',(-4.05596218814324,13.3852500034686,-5.58255302587488));
#30101=CARTESIAN_POINT('Ctrl Pts',(-2.0279810940716,13.2582500034686,-6.24148402692676));
#30102=CARTESIAN_POINT('Ctrl Pts',(0.,13.1312500034686,-6.90041502797853));
#30103=CARTESIAN_POINT('Ctrl Pts',(2.02798109407148,13.0042500034686,-6.24148402692676));
#30104=CARTESIAN_POINT('Ctrl Pts',(4.05596218814312,12.8772500034686,-5.58255302587488));
#30105=CARTESIAN_POINT('Ctrl Pts',(5.30932343282159,12.7502500034686,-3.85744926888038));
#30106=CARTESIAN_POINT('Ctrl Pts',(6.56268467750003,12.6232500034687,-2.13234551188562));
#30107=CARTESIAN_POINT('Ctrl Pts',(6.56268467749999,12.4962500034686,-5.55111512312578E-14));
#30108=CARTESIAN_POINT('Ctrl Pts',(6.56268467749997,12.3692500034686,2.13234551188562));
#30109=CARTESIAN_POINT('Ctrl Pts',(5.30932343282153,12.2422500034687,3.85744926888026));
#30110=CARTESIAN_POINT('Ctrl Pts',(4.05596218814312,12.1152500034686,5.58255302587488));
#30111=CARTESIAN_POINT('Ctrl Pts',(2.02798109407154,11.9882500034686,6.24148402692665));
#30112=CARTESIAN_POINT('Ctrl Pts',(0.,11.8612500034686,6.90041502797853));
#30113=CARTESIAN_POINT('Ctrl Pts',(-2.02798109407154,11.7342500034686,6.24148402692665));
#30114=CARTESIAN_POINT('Ctrl Pts',(-4.05596218814312,11.6072500034687,5.58255302587488));
#30115=CARTESIAN_POINT('Ctrl Pts',(-5.30932343282153,11.4802500034686,3.85744926888026));
#30116=CARTESIAN_POINT('Ctrl Pts',(-6.56268467749997,11.3532500034686,2.13234551188562));
#30117=CARTESIAN_POINT('Ctrl Pts',(-6.56268467749999,11.2262500034686,-5.55111512312578E-14));
#30118=CARTESIAN_POINT('Ctrl Pts',(-6.56268467750003,11.0992500034686,-2.13234551188562));
#30119=CARTESIAN_POINT('Ctrl Pts',(-5.30932343282159,10.9722500034686,-3.85744926888038));
#30120=CARTESIAN_POINT('Ctrl Pts',(-4.05596218814312,10.8452500034687,-5.58255302587488));
#30121=CARTESIAN_POINT('Ctrl Pts',(-2.0279810940716,10.7182500034686,-6.24148402692676));
#30122=CARTESIAN_POINT('Ctrl Pts',(0.,10.5912500034686,-6.90041502797853));
#30123=CARTESIAN_POINT('Ctrl Pts',(2.0279810940716,10.4642500034686,-6.24148402692676));
#30124=CARTESIAN_POINT('Ctrl Pts',(4.05596218814324,10.3372500034686,-5.58255302587488));
#30125=CARTESIAN_POINT('Ctrl Pts',(5.30932343282153,10.2102500034685,-3.85744926888038));
#30126=CARTESIAN_POINT('Ctrl Pts',(6.56268467749991,10.0832500034686,-2.13234551188562));
#30127=CARTESIAN_POINT('Ctrl Pts',(6.56268467749999,9.95625000346861,-5.55111512312578E-14));
#30128=CARTESIAN_POINT('Ctrl Pts',(6.56268467750008,9.8292500034686,2.13234551188562));
#30129=CARTESIAN_POINT('Ctrl Pts',(5.30932343282164,9.70225000346864,3.85744926888026));
#30130=CARTESIAN_POINT('Ctrl Pts',(4.05596218814312,9.57525000346868,5.58255302587488));
#30131=CARTESIAN_POINT('Ctrl Pts',(2.02798109407154,9.44825000346855,6.24148402692665));
#30132=CARTESIAN_POINT('Ctrl Pts',(0.,9.32125000346853,6.90041502797853));
#30133=CARTESIAN_POINT('Ctrl Pts',(-2.02798109407154,9.19425000346857,6.24148402692665));
#30134=CARTESIAN_POINT('Ctrl Pts',(-4.05596218814312,9.06725000346862,5.58255302587488));
#30135=CARTESIAN_POINT('Ctrl Pts',(-5.30932343282159,8.9402500034686,3.85744926888026));
#30136=CARTESIAN_POINT('Ctrl Pts',(-6.56268467749997,8.81325000346859,2.13234551188562));
#30137=CARTESIAN_POINT('Ctrl Pts',(-6.56268467749999,8.68625000346862,-5.55111512312578E-14));
#30138=CARTESIAN_POINT('Ctrl Pts',(-6.56268467750003,8.55925000346873,-2.13234551188562));
#30139=CARTESIAN_POINT('Ctrl Pts',(-5.30932343282159,8.43225000346859,-3.85744926888038));
#30140=CARTESIAN_POINT('Ctrl Pts',(-4.05596218814312,8.30525000346876,-5.58255302587488));
#30141=CARTESIAN_POINT('Ctrl Pts',(-2.02798109407148,8.17825000346861,-6.24148402692676));
#30142=CARTESIAN_POINT('Ctrl Pts',(0.,8.05125000346861,-6.90041502797853));
#30143=CARTESIAN_POINT('Ctrl Pts',(2.02798109407154,7.92425000346864,-6.24148402692676));
#30144=CARTESIAN_POINT('Ctrl Pts',(4.05596218814312,7.79725000346864,-5.58255302587488));
#30145=CARTESIAN_POINT('Ctrl Pts',(5.30932343282153,7.67025000346866,-3.85744926888038));
#30146=CARTESIAN_POINT('Ctrl Pts',(6.56268467750003,7.5432500034686,-2.13234551188562));
#30147=CARTESIAN_POINT('Ctrl Pts',(6.56268467749999,7.41625000346852,-5.55111512312578E-14));
#30148=CARTESIAN_POINT('Ctrl Pts',(6.56268467749997,7.28925000346863,2.13234551188562));
#30149=CARTESIAN_POINT('Ctrl Pts',(5.30932343282159,7.1622500034686,3.85744926888026));
#30150=CARTESIAN_POINT('Ctrl Pts',(4.05596218814312,7.0352500034686,5.58255302587488));
#30151=CARTESIAN_POINT('Ctrl Pts',(2.02798109407154,6.90825000346851,6.24148402692665));
#30152=CARTESIAN_POINT('Ctrl Pts',(0.,6.78125000346874,6.90041502797853));
#30153=CARTESIAN_POINT('Ctrl Pts',(-2.0279810940716,6.65425000346853,6.24148402692665));
#30154=CARTESIAN_POINT('Ctrl Pts',(-4.05596218814312,6.52725000346859,5.58255302587488));
#30155=CARTESIAN_POINT('Ctrl Pts',(-5.30932343282159,6.40025000346872,3.85744926888026));
#30156=CARTESIAN_POINT('Ctrl Pts',(-6.56268467749997,6.27325000346868,2.13234551188562));
#30157=CARTESIAN_POINT('Ctrl Pts',(-6.56268467749993,6.14625000346863,0.));
#30158=CARTESIAN_POINT('Ctrl Pts',(-6.56268467749991,6.01925000346865,-2.13234551188562));
#30159=CARTESIAN_POINT('Ctrl Pts',(-5.30932343282159,5.8922500034686,-3.85744926888032));
#30160=CARTESIAN_POINT('Ctrl Pts',(-4.05596218814312,5.76525000346862,-5.58255302587488));
#30161=CARTESIAN_POINT('Ctrl Pts',(-2.02798109407154,5.63825000346863,-6.2414840269267));
#30162=CARTESIAN_POINT('Ctrl Pts',(0.,5.5112500034687,-6.90041502797853));
#30163=CARTESIAN_POINT('Ctrl Pts',(2.02798109407154,5.38425000346859,-6.2414840269267));
#30164=CARTESIAN_POINT('Ctrl Pts',(4.05596218814324,5.25725000346861,-5.58255302587488));
#30165=CARTESIAN_POINT('Ctrl Pts',(5.30932343282159,5.13025000346867,-3.85744926888032));
#30166=CARTESIAN_POINT('Ctrl Pts',(6.56268467750003,5.00325000346858,-2.13234551188562));
#30167=CARTESIAN_POINT('Ctrl Pts',(6.56268467749999,4.87625000346864,0.));
#30168=CARTESIAN_POINT('Ctrl Pts',(6.56268467750008,4.74925000346872,2.13234551188562));
#30169=CARTESIAN_POINT('Ctrl Pts',(5.30932343282159,4.62225000346861,3.85744926888032));
#30170=CARTESIAN_POINT('Ctrl Pts',(4.05596218814312,4.49525000346869,5.58255302587488));
#30171=CARTESIAN_POINT('Ctrl Pts',(2.02798109407148,4.36825000346869,6.2414840269267));
#30172=CARTESIAN_POINT('Ctrl Pts',(0.,4.24125000346866,6.90041502797853));
#30173=CARTESIAN_POINT('Ctrl Pts',(-2.0279810940716,4.11425000346871,6.2414840269267));
#30174=CARTESIAN_POINT('Ctrl Pts',(-4.05596218814312,3.98725000346863,5.58255302587488));
#30175=CARTESIAN_POINT('Ctrl Pts',(-5.30932343282159,3.86025000346862,3.85744926888032));
#30176=CARTESIAN_POINT('Ctrl Pts',(-6.56268467749997,3.7332500034686,2.13234551188562));
#30177=CARTESIAN_POINT('Ctrl Pts',(-6.56268467749999,3.60625000346859,0.));
#30178=CARTESIAN_POINT('Ctrl Pts',(-6.56268467750008,3.47925000346862,-2.13234551188562));
#30179=CARTESIAN_POINT('Ctrl Pts',(-5.30932343282159,3.3522500034685,-3.85744926888032));
#30180=CARTESIAN_POINT('Ctrl Pts',(-4.05596218814312,3.22525000346859,-5.58255302587488));
#30181=CARTESIAN_POINT('Ctrl Pts',(-2.02798109407154,3.09825000346858,-6.2414840269267));
#30182=CARTESIAN_POINT('Ctrl Pts',(5.83678785436452E-14,2.97125000346862,
-6.90041502797853));
#30183=CARTESIAN_POINT('Ctrl Pts',(2.02798109407154,2.84425000346861,-6.2414840269267));
#30184=CARTESIAN_POINT('Ctrl Pts',(4.05596218814318,2.71725000346853,-5.58255302587488));
#30185=CARTESIAN_POINT('Ctrl Pts',(5.30932343282159,2.59025000346863,-3.85744926888032));
#30186=CARTESIAN_POINT('Ctrl Pts',(6.56268467750003,2.46325000346861,-2.13234551188562));
#30187=CARTESIAN_POINT('Ctrl Pts',(6.56268467749993,2.3362500034686,0.));
#30188=CARTESIAN_POINT('Ctrl Pts',(6.56268467750003,2.20925000346864,2.13234551188562));
#30189=CARTESIAN_POINT('Ctrl Pts',(5.30932343282159,2.08225000346862,3.85744926888032));
#30190=CARTESIAN_POINT('Ctrl Pts',(4.05596218814324,1.95525000346861,5.58255302587488));
#30191=CARTESIAN_POINT('Ctrl Pts',(2.02798109407148,1.82825000346865,6.2414840269267));
#30192=CARTESIAN_POINT('Ctrl Pts',(1.1673575708729E-13,1.70125000346858,
6.90041502797853));
#30193=CARTESIAN_POINT('Ctrl Pts',(-2.02798109407148,1.57425000346872,6.2414840269267));
#30194=CARTESIAN_POINT('Ctrl Pts',(-4.05596218814306,1.44725000346872,5.58255302587488));
#30195=CARTESIAN_POINT('Ctrl Pts',(-5.30932343282159,1.32025000346858,3.85744926888032));
#30196=CARTESIAN_POINT('Ctrl Pts',(-6.56268467750003,1.19325000346869,2.13234551188562));
#30197=CARTESIAN_POINT('Ctrl Pts',(-6.56268467749999,1.06625000346861,0.));
#30198=CARTESIAN_POINT('Ctrl Pts',(-6.56268467749997,0.939250003468656,
-2.13234551188562));
#30199=CARTESIAN_POINT('Ctrl Pts',(-5.30932343282164,0.812250003468629,
-3.85744926888032));
#30200=CARTESIAN_POINT('Ctrl Pts',(-4.05596218814312,0.685250003468624,
-5.58255302587488));
#30201=CARTESIAN_POINT('Ctrl Pts',(-2.02798109407154,0.558250003468708,
-6.2414840269267));
#30202=CARTESIAN_POINT('Ctrl Pts',(0.,0.431250003468709,-6.90041502797853));
#30203=CARTESIAN_POINT('Ctrl Pts',(2.02798109407154,0.30425000346862,-6.2414840269267));
#30204=CARTESIAN_POINT('Ctrl Pts',(4.05596218814306,0.177250003468736,-5.58255302587488));
#30205=CARTESIAN_POINT('Ctrl Pts',(5.30932343282159,0.0502500034685882,
-3.85744926888032));
#30206=CARTESIAN_POINT('Ctrl Pts',(6.56268467750003,-0.0767499965312958,
-2.13234551188562));
#30207=CARTESIAN_POINT('Ctrl Pts',(6.56268467749993,-0.203749996531333,
0.));
#30208=CARTESIAN_POINT('Ctrl Pts',(6.56268467749991,-0.330749996531386,
2.13234551188562));
#30209=CARTESIAN_POINT('Ctrl Pts',(5.30932343282159,-0.45774999653142,3.85744926888032));
#30210=CARTESIAN_POINT('Ctrl Pts',(4.05596218814312,-0.584749996531417,
5.58255302587488));
#30211=CARTESIAN_POINT('Ctrl Pts',(2.0279810940716,-0.711749996531397,6.2414840269267));
#30212=CARTESIAN_POINT('Ctrl Pts',(1.3927615077689,-0.751529897683364,6.44787938194943));
#30213=CARTESIAN_POINT('Ctrl Pts',(0.728985515936097,-0.793098111119581,
6.5220710126346));
#30214=CARTESIAN_POINT('Ctrl Pts',(-7.9375000000001,17.0999999999999,-5.55111512312578E-14));
#30215=CARTESIAN_POINT('Ctrl Pts',(-7.93750000000009,16.973,-2.57905008884871));
#30216=CARTESIAN_POINT('Ctrl Pts',(-6.42157239285118,16.846,-4.66554544007153));
#30217=CARTESIAN_POINT('Ctrl Pts',(-4.90564478570231,16.7190000000001,-6.7520407912943));
#30218=CARTESIAN_POINT('Ctrl Pts',(-2.45282239285105,16.592,-7.54901109809286));
#30219=CARTESIAN_POINT('Ctrl Pts',(0.,16.465,-8.34598140489129));
#30220=CARTESIAN_POINT('Ctrl Pts',(2.45282239285116,16.338,-7.54901109809286));
#30221=CARTESIAN_POINT('Ctrl Pts',(4.90564478570226,16.2110000000001,-6.7520407912943));
#30222=CARTESIAN_POINT('Ctrl Pts',(6.42157239285113,16.084,-4.66554544007153));
#30223=CARTESIAN_POINT('Ctrl Pts',(7.93750000000003,15.9569999999999,-2.57905008884871));
#30224=CARTESIAN_POINT('Ctrl Pts',(7.93749999999999,15.83,-5.55111512312578E-14));
#30225=CARTESIAN_POINT('Ctrl Pts',(7.93750000000009,15.703,2.57905008884871));
#30226=CARTESIAN_POINT('Ctrl Pts',(6.42157239285113,15.576,4.66554544007142));
#30227=CARTESIAN_POINT('Ctrl Pts',(4.90564478570226,15.449,6.7520407912943));
#30228=CARTESIAN_POINT('Ctrl Pts',(2.45282239285122,15.3220000000001,7.54901109809275));
#30229=CARTESIAN_POINT('Ctrl Pts',(0.,15.195,8.34598140489129));
#30230=CARTESIAN_POINT('Ctrl Pts',(-2.45282239285116,15.068,7.54901109809275));
#30231=CARTESIAN_POINT('Ctrl Pts',(-4.90564478570231,14.9410000000001,6.7520407912943));
#30232=CARTESIAN_POINT('Ctrl Pts',(-6.42157239285118,14.8140000000001,4.66554544007142));
#30233=CARTESIAN_POINT('Ctrl Pts',(-7.93750000000003,14.687,2.57905008884871));
#30234=CARTESIAN_POINT('Ctrl Pts',(-7.9375000000001,14.56,-5.55111512312578E-14));
#30235=CARTESIAN_POINT('Ctrl Pts',(-7.93749999999997,14.4330000000001,-2.57905008884871));
#30236=CARTESIAN_POINT('Ctrl Pts',(-6.42157239285124,14.306,-4.66554544007153));
#30237=CARTESIAN_POINT('Ctrl Pts',(-4.90564478570231,14.179,-6.7520407912943));
#30238=CARTESIAN_POINT('Ctrl Pts',(-2.45282239285111,14.052,-7.54901109809286));
#30239=CARTESIAN_POINT('Ctrl Pts',(0.,13.9250000000001,-8.34598140489129));
#30240=CARTESIAN_POINT('Ctrl Pts',(2.45282239285116,13.798,-7.54901109809286));
#30241=CARTESIAN_POINT('Ctrl Pts',(4.90564478570226,13.671,-6.7520407912943));
#30242=CARTESIAN_POINT('Ctrl Pts',(6.42157239285113,13.544,-4.66554544007153));
#30243=CARTESIAN_POINT('Ctrl Pts',(7.93750000000003,13.4170000000001,-2.57905008884871));
#30244=CARTESIAN_POINT('Ctrl Pts',(7.93749999999999,13.29,-5.55111512312578E-14));
#30245=CARTESIAN_POINT('Ctrl Pts',(7.93750000000003,13.1630000000001,2.57905008884871));
#30246=CARTESIAN_POINT('Ctrl Pts',(6.42157239285113,13.036,4.66554544007142));
#30247=CARTESIAN_POINT('Ctrl Pts',(4.90564478570226,12.9090000000001,6.7520407912943));
#30248=CARTESIAN_POINT('Ctrl Pts',(2.45282239285116,12.7820000000001,7.54901109809275));
#30249=CARTESIAN_POINT('Ctrl Pts',(0.,12.6550000000001,8.34598140489129));
#30250=CARTESIAN_POINT('Ctrl Pts',(-2.45282239285116,12.528,7.54901109809275));
#30251=CARTESIAN_POINT('Ctrl Pts',(-4.9056447857022,12.401,6.7520407912943));
#30252=CARTESIAN_POINT('Ctrl Pts',(-6.42157239285124,12.274,4.66554544007142));
#30253=CARTESIAN_POINT('Ctrl Pts',(-7.93750000000003,12.1470000000001,2.57905008884871));
#30254=CARTESIAN_POINT('Ctrl Pts',(-7.9375000000001,12.0200000000001,-5.55111512312578E-14));
#30255=CARTESIAN_POINT('Ctrl Pts',(-7.93749999999997,11.8930000000001,-2.57905008884871));
#30256=CARTESIAN_POINT('Ctrl Pts',(-6.42157239285124,11.766,-4.66554544007153));
#30257=CARTESIAN_POINT('Ctrl Pts',(-4.90564478570231,11.639,-6.7520407912943));
#30258=CARTESIAN_POINT('Ctrl Pts',(-2.45282239285111,11.512,-7.54901109809286));
#30259=CARTESIAN_POINT('Ctrl Pts',(1.1673575708729E-13,11.3850000000001,
-8.34598140489129));
#30260=CARTESIAN_POINT('Ctrl Pts',(2.45282239285116,11.258,-7.54901109809286));
#30261=CARTESIAN_POINT('Ctrl Pts',(4.90564478570231,11.131,-6.7520407912943));
#30262=CARTESIAN_POINT('Ctrl Pts',(6.42157239285113,11.004,-4.66554544007153));
#30263=CARTESIAN_POINT('Ctrl Pts',(7.93750000000003,10.877,-2.57905008884871));
#30264=CARTESIAN_POINT('Ctrl Pts',(7.93749999999999,10.75,-5.55111512312578E-14));
#30265=CARTESIAN_POINT('Ctrl Pts',(7.93749999999991,10.623,2.57905008884871));
#30266=CARTESIAN_POINT('Ctrl Pts',(6.42157239285113,10.496,4.66554544007142));
#30267=CARTESIAN_POINT('Ctrl Pts',(4.90564478570237,10.369,6.7520407912943));
#30268=CARTESIAN_POINT('Ctrl Pts',(2.45282239285116,10.242,7.54901109809275));
#30269=CARTESIAN_POINT('Ctrl Pts',(1.1673575708729E-13,10.115,8.34598140489129));
#30270=CARTESIAN_POINT('Ctrl Pts',(-2.45282239285105,9.988,7.54901109809275));
#30271=CARTESIAN_POINT('Ctrl Pts',(-4.90564478570231,9.86100000000001,6.7520407912943));
#30272=CARTESIAN_POINT('Ctrl Pts',(-6.42157239285124,9.73400000000002,4.66554544007142));
#30273=CARTESIAN_POINT('Ctrl Pts',(-7.93750000000003,9.60699999999999,2.57905008884871));
#30274=CARTESIAN_POINT('Ctrl Pts',(-7.93750000000004,9.48000000000004,-5.55111512312578E-14));
#30275=CARTESIAN_POINT('Ctrl Pts',(-7.93749999999997,9.35300000000001,-2.57905008884871));
#30276=CARTESIAN_POINT('Ctrl Pts',(-6.42157239285124,9.22600000000001,-4.66554544007153));
#30277=CARTESIAN_POINT('Ctrl Pts',(-4.9056447857022,9.09899999999998,-6.7520407912943));
#30278=CARTESIAN_POINT('Ctrl Pts',(-2.45282239285116,8.97200000000004,-7.54901109809286));
#30279=CARTESIAN_POINT('Ctrl Pts',(0.,8.84500000000001,-8.34598140489129));
#30280=CARTESIAN_POINT('Ctrl Pts',(2.45282239285122,8.718,-7.54901109809286));
#30281=CARTESIAN_POINT('Ctrl Pts',(4.9056447857022,8.59100000000003,-6.7520407912943));
#30282=CARTESIAN_POINT('Ctrl Pts',(6.42157239285113,8.46399999999992,-4.66554544007153));
#30283=CARTESIAN_POINT('Ctrl Pts',(7.93750000000009,8.33700000000012,-2.57905008884871));
#30284=CARTESIAN_POINT('Ctrl Pts',(7.93749999999999,8.21,-5.55111512312578E-14));
#30285=CARTESIAN_POINT('Ctrl Pts',(7.93750000000003,8.08299999999997,2.57905008884871));
#30286=CARTESIAN_POINT('Ctrl Pts',(6.42157239285107,7.95600000000002,4.66554544007142));
#30287=CARTESIAN_POINT('Ctrl Pts',(4.90564478570237,7.829,6.7520407912943));
#30288=CARTESIAN_POINT('Ctrl Pts',(2.45282239285116,7.70199999999999,7.54901109809275));
#30289=CARTESIAN_POINT('Ctrl Pts',(0.,7.57500000000008,8.34598140489129));
#30290=CARTESIAN_POINT('Ctrl Pts',(-2.45282239285105,7.44800000000001,7.54901109809275));
#30291=CARTESIAN_POINT('Ctrl Pts',(-4.90564478570231,7.32100000000005,6.7520407912943));
#30292=CARTESIAN_POINT('Ctrl Pts',(-6.42157239285124,7.19399999999998,4.66554544007142));
#30293=CARTESIAN_POINT('Ctrl Pts',(-7.93749999999991,7.06700000000008,2.57905008884871));
#30294=CARTESIAN_POINT('Ctrl Pts',(-7.93749999999999,6.94,-5.55111512312578E-14));
#30295=CARTESIAN_POINT('Ctrl Pts',(-7.93749999999997,6.8130000000001,-2.57905008884871));
#30296=CARTESIAN_POINT('Ctrl Pts',(-6.42157239285113,6.68600000000008,-4.66554544007153));
#30297=CARTESIAN_POINT('Ctrl Pts',(-4.90564478570231,6.55900000000001,-6.7520407912943));
#30298=CARTESIAN_POINT('Ctrl Pts',(-2.45282239285116,6.4320000000001,-7.54901109809286));
#30299=CARTESIAN_POINT('Ctrl Pts',(-1.1673575708729E-13,6.3050000000001,
-8.34598140489129));
#30300=CARTESIAN_POINT('Ctrl Pts',(2.45282239285116,6.17799999999996,-7.54901109809286));
#30301=CARTESIAN_POINT('Ctrl Pts',(4.90564478570231,6.05100000000001,-6.7520407912943));
#30302=CARTESIAN_POINT('Ctrl Pts',(6.42157239285107,5.92399999999999,-4.66554544007147));
#30303=CARTESIAN_POINT('Ctrl Pts',(7.93749999999997,5.79700000000004,-2.57905008884871));
#30304=CARTESIAN_POINT('Ctrl Pts',(7.93749999999999,5.66999999999995,0.));
#30305=CARTESIAN_POINT('Ctrl Pts',(7.93750000000003,5.543,2.57905008884871));
#30306=CARTESIAN_POINT('Ctrl Pts',(6.42157239285107,5.41599999999998,4.66554544007147));
#30307=CARTESIAN_POINT('Ctrl Pts',(4.9056447857022,5.28900000000003,6.7520407912943));
#30308=CARTESIAN_POINT('Ctrl Pts',(2.45282239285116,5.16199999999994,7.54901109809281));
#30309=CARTESIAN_POINT('Ctrl Pts',(0.,5.035,8.34598140489129));
#30310=CARTESIAN_POINT('Ctrl Pts',(-2.45282239285111,4.90800000000008,7.54901109809281));
#30311=CARTESIAN_POINT('Ctrl Pts',(-4.90564478570226,4.78099999999997,6.7520407912943));
#30312=CARTESIAN_POINT('Ctrl Pts',(-6.42157239285113,4.65399999999999,4.66554544007147));
#30313=CARTESIAN_POINT('Ctrl Pts',(-7.93750000000003,4.52699999999999,2.57905008884871));
#30314=CARTESIAN_POINT('Ctrl Pts',(-7.93750000000004,4.39999999999996,0.));
#30315=CARTESIAN_POINT('Ctrl Pts',(-7.93750000000003,4.27300000000002,-2.57905008884871));
#30316=CARTESIAN_POINT('Ctrl Pts',(-6.42157239285118,4.14600000000004,-4.66554544007147));
#30317=CARTESIAN_POINT('Ctrl Pts',(-4.9056447857022,4.0190000000001,-6.7520407912943));
#30318=CARTESIAN_POINT('Ctrl Pts',(-2.45282239285116,3.89200000000006,-7.54901109809281));
#30319=CARTESIAN_POINT('Ctrl Pts',(0.,3.76500000000001,-8.34598140489129));
#30320=CARTESIAN_POINT('Ctrl Pts',(2.45282239285116,3.63800000000003,-7.54901109809281));
#30321=CARTESIAN_POINT('Ctrl Pts',(4.90564478570231,3.51100000000004,-6.7520407912943));
#30322=CARTESIAN_POINT('Ctrl Pts',(6.42157239285107,3.38400000000011,-4.66554544007147));
#30323=CARTESIAN_POINT('Ctrl Pts',(7.93749999999997,3.25700000000001,-2.57905008884871));
#30324=CARTESIAN_POINT('Ctrl Pts',(7.93749999999993,3.13000000000002,0.));
#30325=CARTESIAN_POINT('Ctrl Pts',(7.93750000000003,3.00299999999998,2.57905008884871));
#30326=CARTESIAN_POINT('Ctrl Pts',(6.42157239285113,2.87599999999993,4.66554544007147));
#30327=CARTESIAN_POINT('Ctrl Pts',(4.90564478570231,2.74900000000001,6.7520407912943));
#30328=CARTESIAN_POINT('Ctrl Pts',(2.45282239285116,2.62200000000001,7.54901109809281));
#30329=CARTESIAN_POINT('Ctrl Pts',(0.,2.49499999999997,8.34598140489129));
#30330=CARTESIAN_POINT('Ctrl Pts',(-2.45282239285111,2.36800000000004,7.54901109809281));
#30331=CARTESIAN_POINT('Ctrl Pts',(-4.90564478570237,2.241,6.7520407912943));
#30332=CARTESIAN_POINT('Ctrl Pts',(-6.42157239285113,2.114,4.66554544007147));
#30333=CARTESIAN_POINT('Ctrl Pts',(-7.93749999999991,1.98699999999997,2.57905008884871));
#30334=CARTESIAN_POINT('Ctrl Pts',(-7.93750000000004,1.85999999999992,0.));
#30335=CARTESIAN_POINT('Ctrl Pts',(-7.93750000000003,1.733,-2.57905008884871));
#30336=CARTESIAN_POINT('Ctrl Pts',(-6.42157239285118,1.606,-4.66554544007147));
#30337=CARTESIAN_POINT('Ctrl Pts',(-4.90564478570226,1.47900000000002,-6.7520407912943));
#30338=CARTESIAN_POINT('Ctrl Pts',(-2.45282239285116,1.35200000000002,-7.54901109809281));
#30339=CARTESIAN_POINT('Ctrl Pts',(-1.1673575708729E-13,1.22499999999999,
-8.34598140489129));
#30340=CARTESIAN_POINT('Ctrl Pts',(2.45282239285116,1.09799999999999,-7.54901109809281));
#30341=CARTESIAN_POINT('Ctrl Pts',(4.90564478570231,0.971000000000075,-6.7520407912943));
#30342=CARTESIAN_POINT('Ctrl Pts',(6.42157239285113,0.844000000000011,-4.66554544007147));
#30343=CARTESIAN_POINT('Ctrl Pts',(7.93750000000009,0.717000000000044,-2.57905008884871));
#30344=CARTESIAN_POINT('Ctrl Pts',(7.93749999999993,0.589999999999979,0.));
#30345=CARTESIAN_POINT('Ctrl Pts',(7.93750000000003,0.463000000000012,2.57905008884871));
#30346=CARTESIAN_POINT('Ctrl Pts',(6.42157239285113,0.336000000000003,4.66554544007147));
#30347=CARTESIAN_POINT('Ctrl Pts',(4.90564478570231,0.208999999999922,6.7520407912943));
#30348=CARTESIAN_POINT('Ctrl Pts',(2.45282239285111,0.082000000000082,7.54901109809281));
#30349=CARTESIAN_POINT('Ctrl Pts',(1.68453079969211,0.0422200988480285,
7.79864416916032));
#30350=CARTESIAN_POINT('Ctrl Pts',(0.881700526094189,0.000651885411683749,
7.88837818770657));
#30351=CARTESIAN_POINT('Ctrl Pts',(6.56268467749999,12.4962500034686,-5.55111512312578E-14));
#30352=CARTESIAN_POINT('Ctrl Pts',(6.56268467749997,12.3692500034686,2.13234551188562));
#30353=CARTESIAN_POINT('Ctrl Pts',(5.30932343282153,12.2422500034687,3.85744926888026));
#30354=CARTESIAN_POINT('Ctrl Pts',(4.05596218814312,12.1152500034686,5.58255302587488));
#30355=CARTESIAN_POINT('Ctrl Pts',(2.02798109407154,11.9882500034686,6.24148402692665));
#30356=CARTESIAN_POINT('Ctrl Pts',(0.,11.8612500034686,6.90041502797853));
#30357=CARTESIAN_POINT('Ctrl Pts',(-2.02798109407154,11.7342500034686,6.24148402692665));
#30358=CARTESIAN_POINT('Ctrl Pts',(-4.05596218814312,11.6072500034687,5.58255302587488));
#30359=CARTESIAN_POINT('Ctrl Pts',(-5.30932343282153,11.4802500034686,3.85744926888026));
#30360=CARTESIAN_POINT('Ctrl Pts',(-6.56268467749997,11.3532500034686,2.13234551188562));
#30361=CARTESIAN_POINT('Ctrl Pts',(-6.56268467749999,11.2262500034686,-5.55111512312578E-14));
#30362=CARTESIAN_POINT('Ctrl Pts',(-6.56268467750003,11.0992500034686,-2.13234551188562));
#30363=CARTESIAN_POINT('Ctrl Pts',(-5.30932343282159,10.9722500034686,-3.85744926888038));
#30364=CARTESIAN_POINT('Ctrl Pts',(-4.05596218814312,10.8452500034687,-5.58255302587488));
#30365=CARTESIAN_POINT('Ctrl Pts',(-2.0279810940716,10.7182500034686,-6.24148402692676));
#30366=CARTESIAN_POINT('Ctrl Pts',(0.,10.5912500034686,-6.90041502797853));
#30367=CARTESIAN_POINT('Ctrl Pts',(2.0279810940716,10.4642500034686,-6.24148402692676));
#30368=CARTESIAN_POINT('Ctrl Pts',(4.05596218814324,10.3372500034686,-5.58255302587488));
#30369=CARTESIAN_POINT('Ctrl Pts',(5.30932343282153,10.2102500034685,-3.85744926888038));
#30370=CARTESIAN_POINT('Ctrl Pts',(6.56268467749991,10.0832500034686,-2.13234551188562));
#30371=CARTESIAN_POINT('Ctrl Pts',(6.56268467749999,9.95625000346861,-5.55111512312578E-14));
#30372=CARTESIAN_POINT('Origin',(-3.44169137633799E-14,15.9887500034686,
-8.78459658321108E-14));
#30373=CARTESIAN_POINT('Ctrl Pts',(6.56268467749999,11.8612500034686,-5.55111512312578E-14));
#30374=CARTESIAN_POINT('Ctrl Pts',(6.56268467750003,11.7342500034686,2.13234551188562));
#30375=CARTESIAN_POINT('Ctrl Pts',(5.30932343282153,11.6072500034686,3.85744926888026));
#30376=CARTESIAN_POINT('Ctrl Pts',(4.05596218814324,11.4802500034687,5.58255302587488));
#30377=CARTESIAN_POINT('Ctrl Pts',(2.02798109407154,11.3532500034686,6.24148402692665));
#30378=CARTESIAN_POINT('Ctrl Pts',(1.1673575708729E-13,11.2262500034686,
6.90041502797853));
#30379=CARTESIAN_POINT('Ctrl Pts',(-2.02798109407154,11.0992500034686,6.24148402692665));
#30380=CARTESIAN_POINT('Ctrl Pts',(-4.05596218814306,10.9722500034686,5.58255302587488));
#30381=CARTESIAN_POINT('Ctrl Pts',(-5.30932343282153,10.8452500034686,3.85744926888026));
#30382=CARTESIAN_POINT('Ctrl Pts',(-6.56268467750003,10.7182500034686,2.13234551188562));
#30383=CARTESIAN_POINT('Ctrl Pts',(-6.56268467749999,10.5912500034687,-5.55111512312578E-14));
#30384=CARTESIAN_POINT('Ctrl Pts',(-6.56268467749997,10.4642500034686,-2.13234551188562));
#30385=CARTESIAN_POINT('Ctrl Pts',(-5.30932343282159,10.3372500034685,-3.85744926888038));
#30386=CARTESIAN_POINT('Ctrl Pts',(-4.05596218814318,10.2102500034686,-5.58255302587488));
#30387=CARTESIAN_POINT('Ctrl Pts',(-2.0279810940716,10.0832500034686,-6.24148402692676));
#30388=CARTESIAN_POINT('Ctrl Pts',(1.1673575708729E-13,9.95625000346861,
-6.90041502797853));
#30389=CARTESIAN_POINT('Ctrl Pts',(2.0279810940716,9.82925000346868,-6.24148402692676));
#30390=CARTESIAN_POINT('Ctrl Pts',(4.05596218814306,9.70225000346858,-5.58255302587488));
#30391=CARTESIAN_POINT('Ctrl Pts',(5.30932343282153,9.57525000346865,-3.85744926888038));
#30392=CARTESIAN_POINT('Ctrl Pts',(6.56268467749997,9.4482500034686,-2.13234551188562));
#30393=CARTESIAN_POINT('Ctrl Pts',(6.56268467749999,9.32125000346862,-5.55111512312578E-14));
#30394=CARTESIAN_POINT('Ctrl Pts',(-7.9375000000001,14.8775000069372,-5.55111512312578E-14));
#30395=CARTESIAN_POINT('Ctrl Pts',(-7.93750000000003,14.7505000069373,-2.57905008884871));
#30396=CARTESIAN_POINT('Ctrl Pts',(-6.42157239285124,14.6235000069372,-4.66554544007153));
#30397=CARTESIAN_POINT('Ctrl Pts',(-4.90564478570237,14.4965000069372,-6.7520407912943));
#30398=CARTESIAN_POINT('Ctrl Pts',(-2.45282239285111,14.3695000069372,-7.54901109809286));
#30399=CARTESIAN_POINT('Ctrl Pts',(0.,14.2425000069373,-8.34598140489129));
#30400=CARTESIAN_POINT('Ctrl Pts',(2.45282239285116,14.1155000069372,-7.54901109809286));
#30401=CARTESIAN_POINT('Ctrl Pts',(4.90564478570231,13.9885000069372,-6.7520407912943));
#30402=CARTESIAN_POINT('Ctrl Pts',(6.42157239285113,13.8615000069372,-4.66554544007153));
#30403=CARTESIAN_POINT('Ctrl Pts',(7.93749999999997,13.7345000069373,-2.57905008884871));
#30404=CARTESIAN_POINT('Ctrl Pts',(7.93749999999999,13.6075000069373,-5.55111512312578E-14));
#30405=CARTESIAN_POINT('Ctrl Pts',(7.93749999999997,13.4805000069373,2.57905008884871));
#30406=CARTESIAN_POINT('Ctrl Pts',(6.42157239285113,13.3535000069373,4.66554544007142));
#30407=CARTESIAN_POINT('Ctrl Pts',(4.90564478570231,13.2265000069373,6.7520407912943));
#30408=CARTESIAN_POINT('Ctrl Pts',(2.45282239285116,13.0995000069373,7.54901109809275));
#30409=CARTESIAN_POINT('Ctrl Pts',(0.,12.9725000069372,8.34598140489129));
#30410=CARTESIAN_POINT('Ctrl Pts',(-2.45282239285105,12.8455000069373,7.54901109809275));
#30411=CARTESIAN_POINT('Ctrl Pts',(-4.90564478570226,12.7185000069372,6.7520407912943));
#30412=CARTESIAN_POINT('Ctrl Pts',(-6.42157239285124,12.5915000069373,4.66554544007142));
#30413=CARTESIAN_POINT('Ctrl Pts',(-7.93749999999997,12.4645000069372,2.57905008884871));
#30414=CARTESIAN_POINT('Ctrl Pts',(-7.93750000000004,12.3375000069372,-5.55111512312578E-14));
#30415=CARTESIAN_POINT('Ctrl Pts',(-7.93750000000003,12.2105000069372,-2.57905008884871));
#30416=CARTESIAN_POINT('Ctrl Pts',(-6.42157239285113,12.0835000069371,-4.66554544007153));
#30417=CARTESIAN_POINT('Ctrl Pts',(-4.90564478570226,11.9565000069372,-6.7520407912943));
#30418=CARTESIAN_POINT('Ctrl Pts',(-2.45282239285111,11.8295000069372,-7.54901109809286));
#30419=CARTESIAN_POINT('Ctrl Pts',(0.,11.7025000069372,-8.34598140489129));
#30420=CARTESIAN_POINT('Ctrl Pts',(2.45282239285122,11.5755000069372,-7.54901109809286));
#30421=CARTESIAN_POINT('Ctrl Pts',(4.90564478570226,11.4485000069373,-6.7520407912943));
#30422=CARTESIAN_POINT('Ctrl Pts',(6.42157239285113,11.3215000069372,-4.66554544007153));
#30423=CARTESIAN_POINT('Ctrl Pts',(7.93750000000003,11.1945000069372,-2.57905008884871));
#30424=CARTESIAN_POINT('Ctrl Pts',(7.93749999999999,11.0675000069372,-5.55111512312578E-14));
#30425=CARTESIAN_POINT('Ctrl Pts',(7.93750000000009,10.9405000069372,2.57905008884871));
#30426=CARTESIAN_POINT('Ctrl Pts',(6.42157239285113,10.8135000069373,4.66554544007142));
#30427=CARTESIAN_POINT('Ctrl Pts',(4.90564478570231,10.6865000069372,6.7520407912943));
#30428=CARTESIAN_POINT('Ctrl Pts',(2.45282239285116,10.5595000069372,7.54901109809275));
#30429=CARTESIAN_POINT('Ctrl Pts',(0.,10.4325000069372,8.34598140489129));
#30430=CARTESIAN_POINT('Ctrl Pts',(-2.45282239285105,10.3055000069373,7.54901109809275));
#30431=CARTESIAN_POINT('Ctrl Pts',(-4.90564478570231,10.1785000069373,6.7520407912943));
#30432=CARTESIAN_POINT('Ctrl Pts',(-6.42157239285124,10.0515000069372,4.66554544007142));
#30433=CARTESIAN_POINT('Ctrl Pts',(-7.93749999999997,9.92450000693731,2.57905008884871));
#30434=CARTESIAN_POINT('Ctrl Pts',(-7.93749999999999,9.7975000069373,-5.55111512312578E-14));
#30435=CARTESIAN_POINT('Ctrl Pts',(-7.93749999999991,9.67050000693722,-2.57905008884871));
#30436=CARTESIAN_POINT('Ctrl Pts',(-6.42157239285113,9.54350000693721,-4.66554544007153));
#30437=CARTESIAN_POINT('Ctrl Pts',(-4.90564478570226,9.41650000693719,-6.7520407912943));
#30438=CARTESIAN_POINT('Ctrl Pts',(-2.45282239285116,9.28950000693724,-7.54901109809286));
#30439=CARTESIAN_POINT('Ctrl Pts',(0.,9.16250000693733,-8.34598140489129));
#30440=CARTESIAN_POINT('Ctrl Pts',(2.45282239285116,9.03550000693709,-7.54901109809286));
#30441=CARTESIAN_POINT('Ctrl Pts',(4.90564478570237,8.90850000693724,-6.7520407912943));
#30442=CARTESIAN_POINT('Ctrl Pts',(6.42157239285113,8.78150000693712,-4.66554544007153));
#30443=CARTESIAN_POINT('Ctrl Pts',(7.93750000000003,8.65450000693732,-2.57905008884871));
#30444=CARTESIAN_POINT('Ctrl Pts',(7.93749999999999,8.52750000693719,-5.55111512312578E-14));
#30445=CARTESIAN_POINT('Ctrl Pts',(7.93749999999997,8.40050000693729,2.57905008884871));
#30446=CARTESIAN_POINT('Ctrl Pts',(6.42157239285113,8.27350000693722,4.66554544007142));
#30447=CARTESIAN_POINT('Ctrl Pts',(4.90564478570231,8.14650000693721,6.7520407912943));
#30448=CARTESIAN_POINT('Ctrl Pts',(2.45282239285116,8.01950000693724,7.54901109809275));
#30449=CARTESIAN_POINT('Ctrl Pts',(1.1673575708729E-13,7.89250000693723,
8.34598140489129));
#30450=CARTESIAN_POINT('Ctrl Pts',(-2.45282239285111,7.76550000693721,7.54901109809275));
#30451=CARTESIAN_POINT('Ctrl Pts',(-4.90564478570231,7.6385000069372,6.7520407912943));
#30452=CARTESIAN_POINT('Ctrl Pts',(-6.42157239285113,7.51150000693718,4.66554544007142));
#30453=CARTESIAN_POINT('Ctrl Pts',(-7.93749999999997,7.38450000693723,2.57905008884871));
#30454=CARTESIAN_POINT('Ctrl Pts',(-7.93749999999999,7.2575000069372,-5.55111512312578E-14));
#30455=CARTESIAN_POINT('Ctrl Pts',(-7.93750000000003,7.13050000693725,-2.57905008884871));
#30456=CARTESIAN_POINT('Ctrl Pts',(-6.42157239285113,7.00350000693733,-4.66554544007153));
#30457=CARTESIAN_POINT('Ctrl Pts',(-4.90564478570231,6.87650000693734,-6.7520407912943));
#30458=CARTESIAN_POINT('Ctrl Pts',(-2.45282239285116,6.74950000693719,-7.54901109809286));
#30459=CARTESIAN_POINT('Ctrl Pts',(0.,6.62250000693725,-8.34598140489129));
#30460=CARTESIAN_POINT('Ctrl Pts',(2.45282239285116,6.49550000693722,-7.54901109809286));
#30461=CARTESIAN_POINT('Ctrl Pts',(4.90564478570226,6.36850000693716,-6.7520407912943));
#30462=CARTESIAN_POINT('Ctrl Pts',(6.42157239285107,6.24150000693724,-4.66554544007153));
#30463=CARTESIAN_POINT('Ctrl Pts',(7.93749999999991,6.11450000693724,-2.57905008884871));
#30464=CARTESIAN_POINT('Ctrl Pts',(7.93749999999993,5.98750000693721,0.));
#30465=CARTESIAN_POINT('Ctrl Pts',(7.93750000000009,5.86050000693721,2.57905008884871));
#30466=CARTESIAN_POINT('Ctrl Pts',(6.42157239285118,5.73350000693723,4.66554544007147));
#30467=CARTESIAN_POINT('Ctrl Pts',(4.90564478570226,5.60650000693724,6.7520407912943));
#30468=CARTESIAN_POINT('Ctrl Pts',(2.45282239285116,5.4795000069372,7.54901109809281));
#30469=CARTESIAN_POINT('Ctrl Pts',(0.,5.35250000693721,8.34598140489129));
#30470=CARTESIAN_POINT('Ctrl Pts',(-2.45282239285111,5.22550000693722,7.54901109809281));
#30471=CARTESIAN_POINT('Ctrl Pts',(-4.90564478570231,5.09850000693718,6.7520407912943));
#30472=CARTESIAN_POINT('Ctrl Pts',(-6.42157239285113,4.97150000693714,4.66554544007147));
#30473=CARTESIAN_POINT('Ctrl Pts',(-7.93749999999997,4.8445000069372,2.57905008884871));
#30474=CARTESIAN_POINT('Ctrl Pts',(-7.93750000000004,4.71750000693721,0.));
#30475=CARTESIAN_POINT('Ctrl Pts',(-7.93749999999997,4.59050000693723,-2.57905008884871));
#30476=CARTESIAN_POINT('Ctrl Pts',(-6.42157239285118,4.46350000693724,-4.66554544007147));
#30477=CARTESIAN_POINT('Ctrl Pts',(-4.90564478570231,4.33650000693731,-6.7520407912943));
#30478=CARTESIAN_POINT('Ctrl Pts',(-2.45282239285116,4.20950000693721,-7.54901109809281));
#30479=CARTESIAN_POINT('Ctrl Pts',(0.,4.08250000693722,-8.34598140489129));
#30480=CARTESIAN_POINT('Ctrl Pts',(2.45282239285116,3.95550000693728,-7.54901109809281));
#30481=CARTESIAN_POINT('Ctrl Pts',(4.90564478570237,3.82850000693731,-6.7520407912943));
#30482=CARTESIAN_POINT('Ctrl Pts',(6.42157239285118,3.7015000069372,-4.66554544007147));
#30483=CARTESIAN_POINT('Ctrl Pts',(7.93750000000003,3.57450000693722,-2.57905008884871));
#30484=CARTESIAN_POINT('Ctrl Pts',(7.93750000000004,3.44750000693711,0.));
#30485=CARTESIAN_POINT('Ctrl Pts',(7.93750000000003,3.32050000693719,2.57905008884871));
#30486=CARTESIAN_POINT('Ctrl Pts',(6.42157239285113,3.19350000693719,4.66554544007147));
#30487=CARTESIAN_POINT('Ctrl Pts',(4.90564478570226,3.06650000693721,6.7520407912943));
#30488=CARTESIAN_POINT('Ctrl Pts',(2.45282239285111,2.93950000693721,7.54901109809281));
#30489=CARTESIAN_POINT('Ctrl Pts',(5.83678785436452E-14,2.81250000693712,
8.34598140489129));
#30490=CARTESIAN_POINT('Ctrl Pts',(-2.45282239285116,2.68550000693712,7.54901109809281));
#30491=CARTESIAN_POINT('Ctrl Pts',(-4.9056447857022,2.55850000693721,6.7520407912943));
#30492=CARTESIAN_POINT('Ctrl Pts',(-6.42157239285113,2.4315000069372,4.66554544007147));
#30493=CARTESIAN_POINT('Ctrl Pts',(-7.93750000000003,2.30450000693723,2.57905008884871));
#30494=CARTESIAN_POINT('Ctrl Pts',(-7.9375000000001,2.17750000693717,0.));
#30495=CARTESIAN_POINT('Ctrl Pts',(-7.93749999999997,2.05050000693714,-2.57905008884871));
#30496=CARTESIAN_POINT('Ctrl Pts',(-6.42157239285118,1.9235000069372,-4.66554544007147));
#30497=CARTESIAN_POINT('Ctrl Pts',(-4.90564478570231,1.79650000693723,-6.7520407912943));
#30498=CARTESIAN_POINT('Ctrl Pts',(-2.45282239285116,1.66950000693722,-7.54901109809281));
#30499=CARTESIAN_POINT('Ctrl Pts',(1.1673575708729E-13,1.54250000693726,
-8.34598140489129));
#30500=CARTESIAN_POINT('Ctrl Pts',(2.45282239285116,1.41550000693724,-7.54901109809281));
#30501=CARTESIAN_POINT('Ctrl Pts',(4.90564478570231,1.28850000693722,-6.7520407912943));
#30502=CARTESIAN_POINT('Ctrl Pts',(6.42157239285113,1.16150000693732,-4.66554544007147));
#30503=CARTESIAN_POINT('Ctrl Pts',(7.93750000000003,1.03450000693719,-2.57905008884871));
#30504=CARTESIAN_POINT('Ctrl Pts',(7.93749999999999,0.907500006937234,0.));
#30505=CARTESIAN_POINT('Ctrl Pts',(7.93749999999991,0.780500006937337,2.57905008884871));
#30506=CARTESIAN_POINT('Ctrl Pts',(6.42157239285113,0.653500006937147,4.66554544007147));
#30507=CARTESIAN_POINT('Ctrl Pts',(4.90564478570237,0.52650000693713,6.7520407912943));
#30508=CARTESIAN_POINT('Ctrl Pts',(2.45282239285122,0.399500006937226,7.54901109809281));
#30509=CARTESIAN_POINT('Ctrl Pts',(1.1673575708729E-13,0.272500006937273,
8.34598140489129));
#30510=CARTESIAN_POINT('Ctrl Pts',(-2.45282239285116,0.145500006937194,
7.54901109809281));
#30511=CARTESIAN_POINT('Ctrl Pts',(-4.90564478570231,0.0185000069371835,
6.7520407912943));
#30512=CARTESIAN_POINT('Ctrl Pts',(-6.42157239285118,-0.108499993062727,
4.66554544007147));
#30513=CARTESIAN_POINT('Ctrl Pts',(-7.93750000000003,-0.23549999306279,
2.57905008884871));
#30514=CARTESIAN_POINT('Ctrl Pts',(-7.9375000000001,-0.362499993062759,
0.));
#30515=CARTESIAN_POINT('Ctrl Pts',(-7.93749999999997,-0.489499993062763,
-2.57905008884871));
#30516=CARTESIAN_POINT('Ctrl Pts',(-6.42157239285124,-0.616499993062791,
-4.66554544007147));
#30517=CARTESIAN_POINT('Ctrl Pts',(-4.90564478570231,-0.743499993062678,
-6.7520407912943));
#30518=CARTESIAN_POINT('Ctrl Pts',(-2.45282239285105,-0.870499993062768,
-7.54901109809281));
#30519=CARTESIAN_POINT('Ctrl Pts',(0.,-0.997499993062768,-8.34598140489129));
#30520=CARTESIAN_POINT('Ctrl Pts',(2.45282239285116,-1.1244999930628,-7.54901109809281));
#30521=CARTESIAN_POINT('Ctrl Pts',(4.9056447857022,-1.2514999930628,-6.7520407912943));
#30522=CARTESIAN_POINT('Ctrl Pts',(6.42157239285113,-1.37849999306278,-4.66554544007147));
#30523=CARTESIAN_POINT('Ctrl Pts',(7.93750000000009,-1.50549999306283,-2.57905008884871));
#30524=CARTESIAN_POINT('Ctrl Pts',(7.93749999999999,-1.6324999930627,0.));
#30525=CARTESIAN_POINT('Ctrl Pts',(7.93750000000003,-1.75949999306275,2.57905008884871));
#30526=CARTESIAN_POINT('Ctrl Pts',(6.42157239285113,-1.88649999306278,4.66554544007147));
#30527=CARTESIAN_POINT('Ctrl Pts',(4.90564478570226,-2.01349999306266,6.7520407912943));
#30528=CARTESIAN_POINT('Ctrl Pts',(2.45282239285116,-2.14049999306282,7.54901109809281));
#30529=CARTESIAN_POINT('Ctrl Pts',(1.68453823965979,-2.18027950899489,7.79864175176826));
#30530=CARTESIAN_POINT('Ctrl Pts',(0.88171591555705,-2.22184731082934,7.88837646757896));
#30531=CARTESIAN_POINT('Ctrl Pts',(-6.56268467749999,15.6712500034686,-5.55111512312578E-14));
#30532=CARTESIAN_POINT('Ctrl Pts',(-6.56268467749997,15.5442500034686,-2.13234551188562));
#30533=CARTESIAN_POINT('Ctrl Pts',(-5.30932343282153,15.4172500034686,-3.85744926888038));
#30534=CARTESIAN_POINT('Ctrl Pts',(-4.05596218814312,15.2902500034686,-5.58255302587488));
#30535=CARTESIAN_POINT('Ctrl Pts',(-2.0279810940716,15.1632500034686,-6.24148402692676));
#30536=CARTESIAN_POINT('Ctrl Pts',(0.,15.0362500034687,-6.90041502797853));
#30537=CARTESIAN_POINT('Ctrl Pts',(2.0279810940716,14.9092500034685,-6.24148402692676));
#30538=CARTESIAN_POINT('Ctrl Pts',(4.05596218814312,14.7822500034687,-5.58255302587488));
#30539=CARTESIAN_POINT('Ctrl Pts',(5.30932343282159,14.6552500034686,-3.85744926888038));
#30540=CARTESIAN_POINT('Ctrl Pts',(6.56268467750003,14.5282500034687,-2.13234551188562));
#30541=CARTESIAN_POINT('Ctrl Pts',(6.56268467749999,14.4012500034687,-5.55111512312578E-14));
#30542=CARTESIAN_POINT('Ctrl Pts',(6.56268467750003,14.2742500034686,2.13234551188562));
#30543=CARTESIAN_POINT('Ctrl Pts',(5.30932343282153,14.1472500034686,3.85744926888026));
#30544=CARTESIAN_POINT('Ctrl Pts',(4.05596218814312,14.0202500034686,5.58255302587488));
#30545=CARTESIAN_POINT('Ctrl Pts',(2.0279810940716,13.8932500034686,6.24148402692665));
#30546=CARTESIAN_POINT('Ctrl Pts',(0.,13.7662500034686,6.90041502797853));
#30547=CARTESIAN_POINT('Ctrl Pts',(-2.02798109407165,13.6392500034685,6.24148402692665));
#30548=CARTESIAN_POINT('Ctrl Pts',(-4.05596218814318,13.5122500034686,5.58255302587488));
#30549=CARTESIAN_POINT('Ctrl Pts',(-5.30932343282153,13.3852500034687,3.85744926888026));
#30550=CARTESIAN_POINT('Ctrl Pts',(-6.56268467750003,13.2582500034686,2.13234551188562));
#30551=CARTESIAN_POINT('Ctrl Pts',(-6.56268467749999,13.1312500034686,-5.55111512312578E-14));
#30552=CARTESIAN_POINT('Ctrl Pts',(-6.56268467749997,13.0042500034686,-2.13234551188562));
#30553=CARTESIAN_POINT('Ctrl Pts',(-5.30932343282153,12.8772500034686,-3.85744926888038));
#30554=CARTESIAN_POINT('Ctrl Pts',(-4.05596218814312,12.7502500034686,-5.58255302587488));
#30555=CARTESIAN_POINT('Ctrl Pts',(-2.0279810940716,12.6232500034686,-6.24148402692676));
#30556=CARTESIAN_POINT('Ctrl Pts',(0.,12.4962500034686,-6.90041502797853));
#30557=CARTESIAN_POINT('Ctrl Pts',(2.0279810940716,12.3692500034686,-6.24148402692676));
#30558=CARTESIAN_POINT('Ctrl Pts',(4.05596218814318,12.2422500034686,-5.58255302587488));
#30559=CARTESIAN_POINT('Ctrl Pts',(5.30932343282159,12.1152500034687,-3.85744926888038));
#30560=CARTESIAN_POINT('Ctrl Pts',(6.56268467749997,11.9882500034686,-2.13234551188562));
#30561=CARTESIAN_POINT('Ctrl Pts',(6.56268467749999,11.8612500034686,-5.55111512312578E-14));
#30562=CARTESIAN_POINT('Ctrl Pts',(6.56268467750003,11.7342500034686,2.13234551188562));
#30563=CARTESIAN_POINT('Ctrl Pts',(5.30932343282153,11.6072500034686,3.85744926888026));
#30564=CARTESIAN_POINT('Ctrl Pts',(4.05596218814324,11.4802500034687,5.58255302587488));
#30565=CARTESIAN_POINT('Ctrl Pts',(2.02798109407154,11.3532500034686,6.24148402692665));
#30566=CARTESIAN_POINT('Ctrl Pts',(1.1673575708729E-13,11.2262500034686,
6.90041502797853));
#30567=CARTESIAN_POINT('Ctrl Pts',(-2.02798109407154,11.0992500034686,6.24148402692665));
#30568=CARTESIAN_POINT('Ctrl Pts',(-4.05596218814306,10.9722500034686,5.58255302587488));
#30569=CARTESIAN_POINT('Ctrl Pts',(-5.30932343282153,10.8452500034686,3.85744926888026));
#30570=CARTESIAN_POINT('Ctrl Pts',(-6.56268467750003,10.7182500034686,2.13234551188562));
#30571=CARTESIAN_POINT('Ctrl Pts',(-6.56268467749999,10.5912500034687,-5.55111512312578E-14));
#30572=CARTESIAN_POINT('Ctrl Pts',(-6.56268467749997,10.4642500034686,-2.13234551188562));
#30573=CARTESIAN_POINT('Ctrl Pts',(-5.30932343282159,10.3372500034685,-3.85744926888038));
#30574=CARTESIAN_POINT('Ctrl Pts',(-4.05596218814318,10.2102500034686,-5.58255302587488));
#30575=CARTESIAN_POINT('Ctrl Pts',(-2.0279810940716,10.0832500034686,-6.24148402692676));
#30576=CARTESIAN_POINT('Ctrl Pts',(1.1673575708729E-13,9.95625000346861,
-6.90041502797853));
#30577=CARTESIAN_POINT('Ctrl Pts',(2.0279810940716,9.82925000346868,-6.24148402692676));
#30578=CARTESIAN_POINT('Ctrl Pts',(4.05596218814306,9.70225000346858,-5.58255302587488));
#30579=CARTESIAN_POINT('Ctrl Pts',(5.30932343282153,9.57525000346865,-3.85744926888038));
#30580=CARTESIAN_POINT('Ctrl Pts',(6.56268467749997,9.4482500034686,-2.13234551188562));
#30581=CARTESIAN_POINT('Ctrl Pts',(6.56268467749999,9.32125000346862,-5.55111512312578E-14));
#30582=CARTESIAN_POINT('Ctrl Pts',(6.56268467750003,9.19425000346858,2.13234551188562));
#30583=CARTESIAN_POINT('Ctrl Pts',(5.30932343282153,9.06725000346864,3.85744926888026));
#30584=CARTESIAN_POINT('Ctrl Pts',(4.05596218814318,8.94025000346872,5.58255302587488));
#30585=CARTESIAN_POINT('Ctrl Pts',(2.02798109407165,8.81325000346872,6.24148402692665));
#30586=CARTESIAN_POINT('Ctrl Pts',(1.1673575708729E-13,8.68625000346869,
6.90041502797853));
#30587=CARTESIAN_POINT('Ctrl Pts',(-2.0279810940716,8.55925000346869,6.24148402692665));
#30588=CARTESIAN_POINT('Ctrl Pts',(-4.05596218814306,8.4322500034686,5.58255302587488));
#30589=CARTESIAN_POINT('Ctrl Pts',(-5.30932343282159,8.3052500034686,3.85744926888026));
#30590=CARTESIAN_POINT('Ctrl Pts',(-6.56268467749991,8.17825000346862,2.13234551188562));
#30591=CARTESIAN_POINT('Ctrl Pts',(-6.56268467749999,8.05125000346868,-5.55111512312578E-14));
#30592=CARTESIAN_POINT('Ctrl Pts',(-6.56268467749997,7.92425000346871,-2.13234551188562));
#30593=CARTESIAN_POINT('Ctrl Pts',(-5.30932343282159,7.79725000346859,-3.85744926888038));
#30594=CARTESIAN_POINT('Ctrl Pts',(-4.05596218814306,7.67025000346873,-5.58255302587488));
#30595=CARTESIAN_POINT('Ctrl Pts',(-2.0279810940716,7.54325000346862,-6.24148402692676));
#30596=CARTESIAN_POINT('Ctrl Pts',(-1.1673575708729E-13,7.41625000346859,
-6.90041502797853));
#30597=CARTESIAN_POINT('Ctrl Pts',(2.02798109407154,7.28925000346869,-6.24148402692676));
#30598=CARTESIAN_POINT('Ctrl Pts',(4.05596218814318,7.16225000346861,-5.58255302587488));
#30599=CARTESIAN_POINT('Ctrl Pts',(5.30932343282153,7.03525000346861,-3.85744926888038));
#30600=CARTESIAN_POINT('Ctrl Pts',(6.56268467750008,6.90825000346864,-2.13234551188562));
#30601=CARTESIAN_POINT('Ctrl Pts',(6.56268467749999,6.78125000346857,-5.55111512312578E-14));
#30602=CARTESIAN_POINT('Ctrl Pts',(6.56268467750003,6.65425000346861,2.13234551188562));
#30603=CARTESIAN_POINT('Ctrl Pts',(5.30932343282148,6.5272500034686,3.85744926888026));
#30604=CARTESIAN_POINT('Ctrl Pts',(4.05596218814318,6.40025000346864,5.58255302587488));
#30605=CARTESIAN_POINT('Ctrl Pts',(2.0279810940716,6.27325000346862,6.24148402692665));
#30606=CARTESIAN_POINT('Ctrl Pts',(-1.1673575708729E-13,6.14625000346872,
6.90041502797853));
#30607=CARTESIAN_POINT('Ctrl Pts',(-2.0279810940716,6.01925000346865,6.2414840269267));
#30608=CARTESIAN_POINT('Ctrl Pts',(-4.05596218814324,5.89225000346851,5.58255302587488));
#30609=CARTESIAN_POINT('Ctrl Pts',(-5.30932343282159,5.76525000346861,3.85744926888032));
#30610=CARTESIAN_POINT('Ctrl Pts',(-6.56268467750003,5.63825000346866,2.13234551188562));
#30611=CARTESIAN_POINT('Ctrl Pts',(-6.56268467750004,5.51125000346864,0.));
#30612=CARTESIAN_POINT('Ctrl Pts',(-6.56268467749997,5.38425000346863,-2.13234551188562));
#30613=CARTESIAN_POINT('Ctrl Pts',(-5.30932343282148,5.25725000346872,-3.85744926888032));
#30614=CARTESIAN_POINT('Ctrl Pts',(-4.05596218814318,5.13025000346865,-5.58255302587488));
#30615=CARTESIAN_POINT('Ctrl Pts',(-2.02798109407165,5.00325000346863,-6.2414840269267));
#30616=CARTESIAN_POINT('Ctrl Pts',(0.,4.87625000346868,-6.90041502797853));
#30617=CARTESIAN_POINT('Ctrl Pts',(2.02798109407154,4.7492500034686,-6.2414840269267));
#30618=CARTESIAN_POINT('Ctrl Pts',(4.05596218814312,4.62225000346859,-5.58255302587488));
#30619=CARTESIAN_POINT('Ctrl Pts',(5.30932343282148,4.49525000346862,-3.85744926888032));
#30620=CARTESIAN_POINT('Ctrl Pts',(6.56268467750008,4.36825000346862,-2.13234551188562));
#30621=CARTESIAN_POINT('Ctrl Pts',(6.5626846775001,4.24125000346864,0.));
#30622=CARTESIAN_POINT('Ctrl Pts',(6.56268467750003,4.1142500034687,2.13234551188562));
#30623=CARTESIAN_POINT('Ctrl Pts',(5.30932343282148,3.98725000346861,3.85744926888032));
#30624=CARTESIAN_POINT('Ctrl Pts',(4.05596218814318,3.86025000346873,5.58255302587488));
#30625=CARTESIAN_POINT('Ctrl Pts',(2.0279810940716,3.73325000346858,6.2414840269267));
#30626=CARTESIAN_POINT('Ctrl Pts',(0.,3.60625000346864,6.90041502797853));
#30627=CARTESIAN_POINT('Ctrl Pts',(-2.0279810940716,3.4792500034686,6.2414840269267));
#30628=CARTESIAN_POINT('Ctrl Pts',(-4.05596218814312,3.35225000346861,5.58255302587488));
#30629=CARTESIAN_POINT('Ctrl Pts',(-5.30932343282159,3.22525000346852,3.85744926888032));
#30630=CARTESIAN_POINT('Ctrl Pts',(-6.56268467749991,3.09825000346869,2.13234551188562));
#30631=CARTESIAN_POINT('Ctrl Pts',(-6.5626846775001,2.9712500034686,0.));
#30632=CARTESIAN_POINT('Ctrl Pts',(-6.56268467750003,2.8442500034686,-2.13234551188562));
#30633=CARTESIAN_POINT('Ctrl Pts',(-5.30932343282148,2.71725000346862,-3.85744926888032));
#30634=CARTESIAN_POINT('Ctrl Pts',(-4.05596218814306,2.59025000346863,-5.58255302587488));
#30635=CARTESIAN_POINT('Ctrl Pts',(-2.02798109407165,2.46325000346864,-6.2414840269267));
#30636=CARTESIAN_POINT('Ctrl Pts',(0.,2.3362500034686,-6.90041502797853));
#30637=CARTESIAN_POINT('Ctrl Pts',(2.02798109407165,2.20925000346861,-6.2414840269267));
#30638=CARTESIAN_POINT('Ctrl Pts',(4.05596218814312,2.08225000346851,-5.58255302587488));
#30639=CARTESIAN_POINT('Ctrl Pts',(5.30932343282148,1.95525000346858,-3.85744926888032));
#30640=CARTESIAN_POINT('Ctrl Pts',(6.56268467749997,1.82825000346865,-2.13234551188562));
#30641=CARTESIAN_POINT('Ctrl Pts',(6.56268467750004,1.7012500034686,0.));
#30642=CARTESIAN_POINT('Ctrl Pts',(6.56268467750014,1.57425000346862,2.13234551188562));
#30643=CARTESIAN_POINT('Ctrl Pts',(5.30932343282148,1.44725000346863,3.85744926888032));
#30644=CARTESIAN_POINT('Ctrl Pts',(4.05596218814318,1.32025000346859,5.58255302587488));
#30645=CARTESIAN_POINT('Ctrl Pts',(2.0279810940716,1.19325000346859,6.2414840269267));
#30646=CARTESIAN_POINT('Ctrl Pts',(0.,1.06625000346873,6.90041502797853));
#30647=CARTESIAN_POINT('Ctrl Pts',(-2.0279810940716,0.939250003468617,6.2414840269267));
#30648=CARTESIAN_POINT('Ctrl Pts',(-4.05596218814312,0.81225000346864,5.58255302587488));
#30649=CARTESIAN_POINT('Ctrl Pts',(-5.30932343282148,0.685250003468529,
3.85744926888032));
#30650=CARTESIAN_POINT('Ctrl Pts',(-6.56268467749997,0.558250003468608,
2.13234551188562));
#30651=CARTESIAN_POINT('Ctrl Pts',(-6.5626846775001,0.431250003468608,0.));
#30652=CARTESIAN_POINT('Ctrl Pts',(-6.56268467750003,0.304250003468635,
-2.13234551188562));
#30653=CARTESIAN_POINT('Ctrl Pts',(-5.30932343282153,0.177250003468632,
-3.85744926888032));
#30654=CARTESIAN_POINT('Ctrl Pts',(-4.05596218814312,0.0502500034686033,
-5.58255302587488));
#30655=CARTESIAN_POINT('Ctrl Pts',(-2.02798109407154,-0.0767499965314,-6.2414840269267));
#30656=CARTESIAN_POINT('Ctrl Pts',(0.,-0.203749996531312,-6.90041502797853));
#30657=CARTESIAN_POINT('Ctrl Pts',(2.0279810940716,-0.330749996531432,-6.2414840269267));
#30658=CARTESIAN_POINT('Ctrl Pts',(4.05596218814312,-0.457749996531285,
-5.58255302587488));
#30659=CARTESIAN_POINT('Ctrl Pts',(5.30932343282148,-0.584749996531464,
-3.85744926888032));
#30660=CARTESIAN_POINT('Ctrl Pts',(6.56268467750003,-0.711749996531317,
-2.13234551188562));
#30661=CARTESIAN_POINT('Ctrl Pts',(6.56268467750004,-0.838749996531385,
0.));
#30662=CARTESIAN_POINT('Ctrl Pts',(6.56268467749997,-0.96574999653129,2.13234551188562));
#30663=CARTESIAN_POINT('Ctrl Pts',(5.30932343282159,-1.09274999653142,3.85744926888032));
#30664=CARTESIAN_POINT('Ctrl Pts',(4.05596218814312,-1.21974999653144,5.58255302587488));
#30665=CARTESIAN_POINT('Ctrl Pts',(2.0279810940716,-1.34674999653139,6.2414840269267));
#30666=CARTESIAN_POINT('Ctrl Pts',(1.39276765909645,-1.38652951246359,6.44787738326189));
#30667=CARTESIAN_POINT('Ctrl Pts',(0.728998239865705,-1.42809731429797,
6.52206959044185));
#30668=CARTESIAN_POINT('Origin',(-9.68966956780948,-5.53100000000001,0.));
#30669=CARTESIAN_POINT('Origin',(100.349250287849,58.0000000000003,-5.55111512312578E-14));
#32880=UNCERTAINTY_MEASURE_WITH_UNIT(LENGTH_MEASURE(0.01),#32904,
'DISTANCE_ACCURACY_VALUE',
'Maximum model space distance between geometric entities at asserted c
onnectivities');
#32886=UNCERTAINTY_MEASURE_WITH_UNIT(LENGTH_MEASURE(0.01),#32904,
'DISTANCE_ACCURACY_VALUE',
'Maximum model space distance between geometric entities at asserted c
onnectivities');
#32897=(
GEOMETRIC_REPRESENTATION_CONTEXT(3)
GLOBAL_UNCERTAINTY_ASSIGNED_CONTEXT((#32880))
GLOBAL_UNIT_ASSIGNED_CONTEXT((#32904,#32906,#32907))
REPRESENTATION_CONTEXT('','3D')
);
#32903=(
GEOMETRIC_REPRESENTATION_CONTEXT(3)
GLOBAL_UNCERTAINTY_ASSIGNED_CONTEXT((#32886))
GLOBAL_UNIT_ASSIGNED_CONTEXT((#32904,#32906,#32907))
REPRESENTATION_CONTEXT('','3D')
);
#32904=(
LENGTH_UNIT()
NAMED_UNIT(*)
SI_UNIT(.MILLI.,.METRE.)
);
#32906=(
NAMED_UNIT(*)
PLANE_ANGLE_UNIT()
SI_UNIT($,.RADIAN.)
);
#32907=(
NAMED_UNIT(*)
SI_UNIT($,.STERADIAN.)
SOLID_ANGLE_UNIT()
);
#32918=SHAPE_DEFINITION_REPRESENTATION(#32934,#33022);
#32934=PRODUCT_DEFINITION_SHAPE('',$,#33039);
#33022=SHAPE_REPRESENTATION('',(#16451),#32897);
#33028=PRODUCT_DEFINITION_CONTEXT('part definition',#33078,'design');
#33039=PRODUCT_DEFINITION('Cover Clamp','Cover Clamp',#33055,#33028);
#33055=PRODUCT_DEFINITION_FORMATION('',$,#33090);
#33078=APPLICATION_CONTEXT(
'Core Data for Automotive Mechanical Design Process');
#33079=PRODUCT_CONTEXT('part definition',#33078,'mechanical');
#33090=PRODUCT('Cover Clamp','Cover Clamp',$,(#33079));
#33100=PRESENTATION_STYLE_ASSIGNMENT((#33106));
#33106=SURFACE_STYLE_USAGE(.BOTH.,#33112);
#33112=SURFACE_SIDE_STYLE('',(#33118));
#33118=SURFACE_STYLE_FILL_AREA(#33124);
#33124=FILL_AREA_STYLE('Opaque(97,158,199)',(#33130));
#33130=FILL_AREA_STYLE_COLOUR('Opaque(97,158,199)',#33136);
#33136=COLOUR_RGB('Opaque(97,158,199)',0.380392156862745,0.619607843137255,
0.780392156862745);
ENDSEC;
END-ISO-10303-21;
